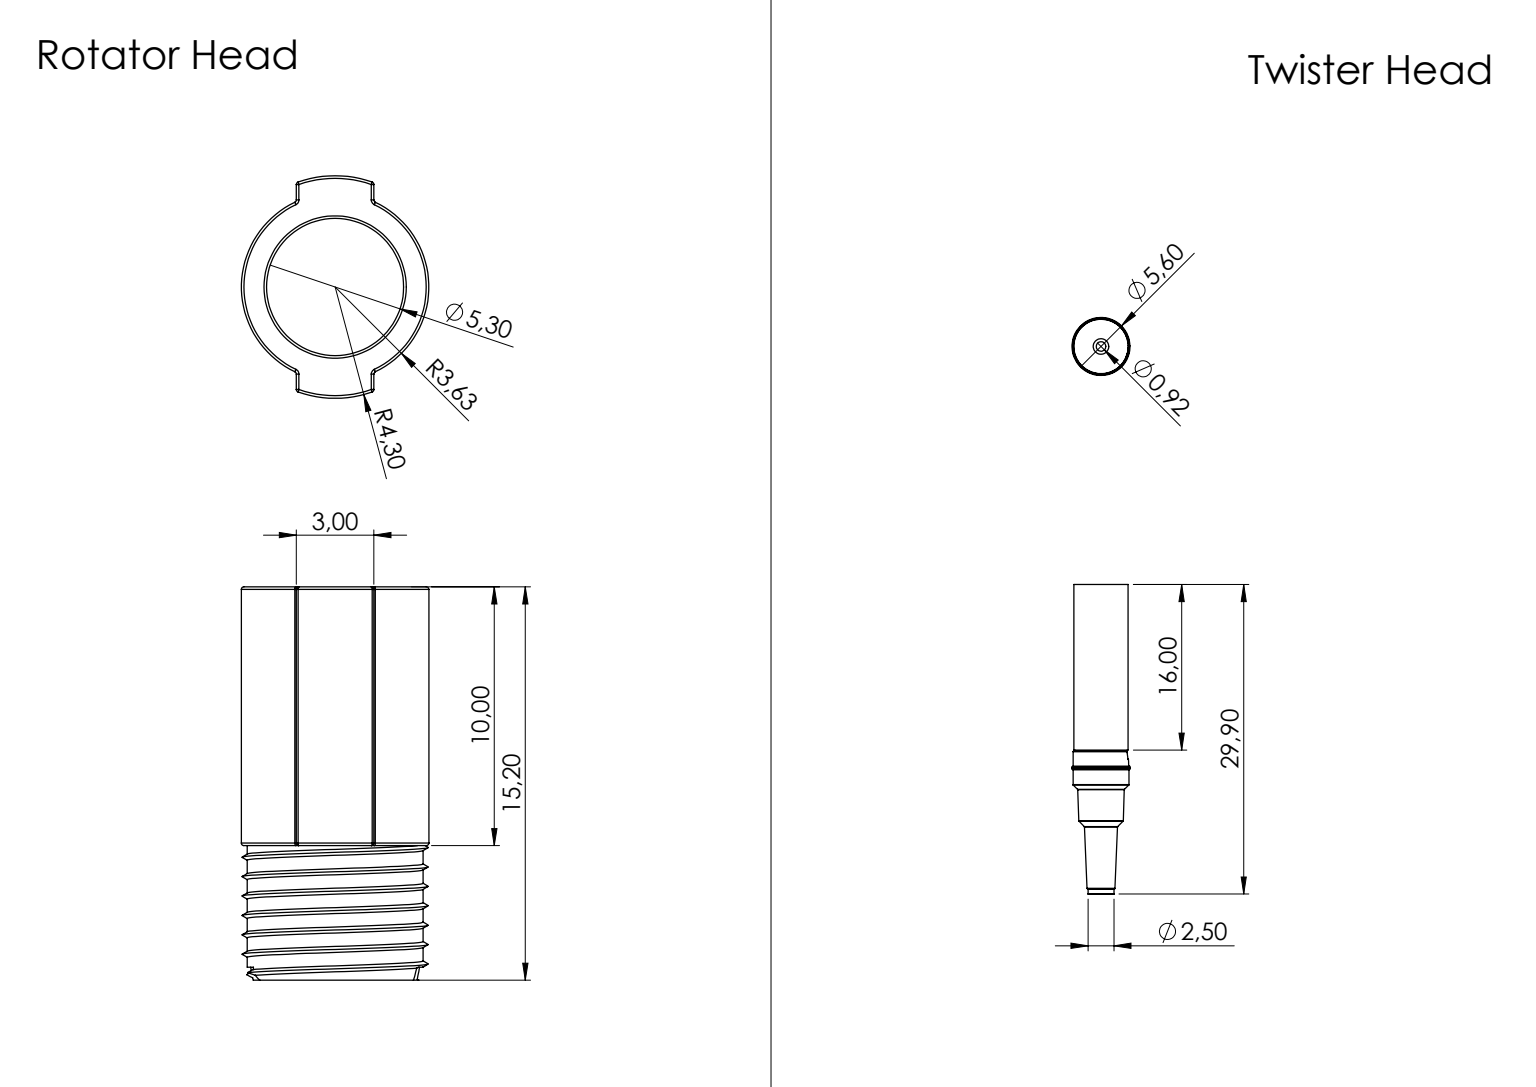
ISO-10303-21;
HEADER;
FILE_DESCRIPTION (('STEP AP214'),
    '1' );
FILE_NAME ('Twister Head.step',
    '2026-10-06T14:00:01',
    ( '' ),
    ( '' ),
    'SwSTEP 2.0',
    'SolidWorks 2020',
    '' );
FILE_SCHEMA (( 'AUTOMOTIVE_DESIGN' ));
ENDSEC;

DATA;
#8=CARTESIAN_POINT ( 'NONE',  ( -62.06147329307218286, -2.678446930503585843, 0.2197408810668839418 ) ) ;
#55=AXIS2_PLACEMENT_3D ( 'NONE', #1109, #22822, #12810 ) ;
#66=VERTEX_POINT ( 'NONE', #447 ) ;
#74=DIRECTION ( 'NONE',  ( -1.000000000000000000, -3.053848253006669023E-16, 2.042510438544995415E-16 ) ) ;
#122=DIRECTION ( 'NONE',  ( 3.002035892788117459E-16, -0.9996898646859343485, -0.02490330187381124480 ) ) ;
#150=CARTESIAN_POINT ( 'NONE',  ( -61.38060080783325390, -2.623833477274086334, -0.6199702340732970995 ) ) ;
#158=DIRECTION ( 'NONE',  ( -1.000000000000000000, -3.053848253006669023E-16, 2.042510438544995415E-16 ) ) ;
#169=DIRECTION ( 'NONE',  ( 0.000000000000000000, -0.9996898646859343485, -0.02490330187381124133 ) ) ;
#190=CARTESIAN_POINT ( 'NONE',  ( -61.37597047653181903, -2.565398393854171122, -0.8228970461733545738 ) ) ;
#193=DIRECTION ( 'NONE',  ( 0.9994629430332292452, 0.03275911391080331414, 0.0008160631928537054542 ) ) ;
#221=ORIENTED_EDGE ( 'NONE', *, *, #12347, .T. ) ;
#253=ORIENTED_EDGE ( 'NONE', *, *, #12134, .F. ) ;
#254=CIRCLE ( 'NONE', #19476, 1.260000000000000231 ) ;
#306=DIRECTION ( 'NONE',  ( 1.000000000000000000, 3.053848253006669023E-16, -2.042510438544995415E-16 ) ) ;
#347=( GEOMETRIC_REPRESENTATION_CONTEXT ( 3 ) GLOBAL_UNCERTAINTY_ASSIGNED_CONTEXT ( ( #22477 ) ) GLOBAL_UNIT_ASSIGNED_CONTEXT ( ( #9070, #19057, #4625 ) ) REPRESENTATION_CONTEXT ( 'NONE', 'WORKASPACE' ) );
#395=EDGE_CURVE ( 'NONE', #29448, #3131, #5108, .T. ) ;
#418=CARTESIAN_POINT ( 'NONE',  ( -73.89999999999997726, 0.4598573377555273400, 0.01145551886195788835 ) ) ;
#427=EDGE_CURVE ( 'NONE', #3316, #29448, #13185, .T. ) ;
#434=ORIENTED_EDGE ( 'NONE', *, *, #19502, .F. ) ;
#447=CARTESIAN_POINT ( 'NONE',  ( -74.39999999999997726, -0.4598573377555325026, -0.01145551886194846360 ) ) ;
#449=FACE_OUTER_BOUND ( 'NONE', #30131, .T. ) ;
#500=CARTESIAN_POINT ( 'NONE',  ( -61.38648119981476015, -2.567347173575106556, -0.8311979704516511136 ) ) ;
#503=CARTESIAN_POINT ( 'NONE',  ( -62.09267578295094125, -2.518691627519130449, 0.1783745650731504706 ) ) ;
#514=CARTESIAN_POINT ( 'NONE',  ( -61.35318038805866081, -2.627373316876406850, 0.4646149771581839505 ) ) ;
#517=CARTESIAN_POINT ( 'NONE',  ( -67.32861504302871936, -2.100022785575387463, -0.05231372570481371970 ) ) ;
#580=CARTESIAN_POINT ( 'NONE',  ( -61.34999999999997300, -2.577403337407089712, -0.5873456857003641618 ) ) ;
#604=LINE ( 'NONE', #19783, #5091 ) ;
#626=CARTESIAN_POINT ( 'NONE',  ( -73.89999999999997726, 0.03361945752964275169, -1.349581317326006946 ) ) ;
#636=CARTESIAN_POINT ( 'NONE',  ( -61.34999999999997300, -2.603451079269508917, 0.4582852780074869736 ) ) ;
#648=CARTESIAN_POINT ( 'NONE',  ( -61.34999999999997300, -2.533482711517546893, -0.7936709607354018869 ) ) ;
#661=CARTESIAN_POINT ( 'NONE',  ( -61.39708522154533199, -2.653109165506343903, 0.5005920380465845865 ) ) ;
#668=ORIENTED_EDGE ( 'NONE', *, *, #22922, .F. ) ;
#680=ORIENTED_EDGE ( 'NONE', *, *, #27825, .F. ) ;
#685=CARTESIAN_POINT ( 'NONE',  ( -67.32861504302871936, -4.287230892216076523E-16, 3.265676834553754426E-15 ) ) ;
#702=CARTESIAN_POINT ( 'NONE',  ( -61.38483210406819524, -2.605333280927485173, 0.7010916910920483858 ) ) ;
#707=DIRECTION ( 'NONE',  ( 3.002035892788117952E-16, -0.9996898646859344595, -0.02490330187381124133 ) ) ;
#761=ORIENTED_EDGE ( 'NONE', *, *, #2889, .F. ) ;
#762=CARTESIAN_POINT ( 'NONE',  ( -61.34999999999997300, -2.456456838093036055, -0.5843327841101846332 ) ) ;
#766=DIRECTION ( 'NONE',  ( 0.7071067811865440200, -0.7068874824028898995, -0.01760929362890773994 ) ) ;
#775=EDGE_CURVE ( 'NONE', #13383, #3831, #22467, .T. ) ;
#782=FACE_OUTER_BOUND ( 'NONE', #5822, .T. ) ;
#784=CARTESIAN_POINT ( 'NONE',  ( -61.39999999999998437, 1.381785979968628826E-15, 2.054751023403646402E-15 ) ) ;
#790=DIRECTION ( 'NONE',  ( 1.000000000000000000, 3.053848253006669023E-16, -2.042510438544995415E-16 ) ) ;
#804=CARTESIAN_POINT ( 'NONE',  ( -67.32861504302871936, 2.100022785575386575, 0.05231372570482049900 ) ) ;
#814=ORIENTED_EDGE ( 'NONE', *, *, #5611, .F. ) ;
#851=EDGE_CURVE ( 'NONE', #22580, #19955, #11332, .T. ) ;
#866=ADVANCED_FACE ( 'NONE', ( #1077 ), #1719, .T. ) ;
#884=ORIENTED_EDGE ( 'NONE', *, *, #22321, .T. ) ;
#886=AXIS2_PLACEMENT_3D ( 'NONE', #30658, #14191, #19131 ) ;
#940=CARTESIAN_POINT ( 'NONE',  ( -62.06710100716626499, -2.504070139480777613, -0.3244344873171103316 ) ) ;
#942=FACE_OUTER_BOUND ( 'NONE', #27423, .T. ) ;
#966=CARTESIAN_POINT ( 'NONE',  ( -61.34999999999997300, -2.606726380931868370, 0.4585432435923214589 ) ) ;
#1017=DIRECTION ( 'NONE',  ( 0.000000000000000000, -0.9996898646859344595, -0.02490330187381124133 ) ) ;
#1069=CARTESIAN_POINT ( 'NONE',  ( -64.28602961791190751, 5.004363292900432036E-16, 2.644225585457161048E-15 ) ) ;
#1077=FACE_OUTER_BOUND ( 'NONE', #10203, .T. ) ;
#1088=CYLINDRICAL_SURFACE ( 'NONE', #11933, 0.7500000000000002220 ) ;
#1104=CYLINDRICAL_SURFACE ( 'NONE', #22252, 2.700000000000000178 ) ;
#1109=CARTESIAN_POINT ( 'NONE',  ( -73.90999999999998238, 1.259609229504275341, 0.03137816036100692790 ) ) ;
#1150=EDGE_CURVE ( 'NONE', #24563, #7611, #31047, .T. ) ;
#1172=CIRCLE ( 'NONE', #8246, 2.700000000000000178 ) ;
#1175=CARTESIAN_POINT ( 'NONE',  ( -61.39062294604998016, -2.605675279217121165, 0.7053491114958538866 ) ) ;
#1179=ORIENTED_EDGE ( 'NONE', *, *, #26385, .F. ) ;
#1180=FACE_OUTER_BOUND ( 'NONE', #3898, .T. ) ;
#1194=AXIS2_PLACEMENT_3D ( 'NONE', #4886, #26749, #24363 ) ;
#1217=ADVANCED_FACE ( 'NONE', ( #3874 ), #26027, .F. ) ;
#1234=ADVANCED_FACE ( 'NONE', ( #1498, #8931 ), #11007, .F. ) ;
#1253=EDGE_CURVE ( 'NONE', #13929, #13516, #22274, .T. ) ;
#1262=DIRECTION ( 'NONE',  ( 0.000000000000000000, 0.9996898646859343485, 0.02490330187381130031 ) ) ;
#1271=CARTESIAN_POINT ( 'NONE',  ( -62.06272861537543406, -2.661683864372939468, -0.3480657431877479668 ) ) ;
#1280=CARTESIAN_POINT ( 'NONE',  ( -60.64999999999998437, -2.458515422985869670, -1.116110171506649040 ) ) ;
#1290=PRESENTATION_STYLE_ASSIGNMENT (( #20643 ) ) ;
#1307=CARTESIAN_POINT ( 'NONE',  ( -64.31974649313019654, 2.248654970328750835, 0.05601630617085266717 ) ) ;
#1309=DIRECTION ( 'NONE',  ( 0.000000000000000000, 0.9996898646859344595, 0.02490330187381124133 ) ) ;
#1310=FACE_OUTER_BOUND ( 'NONE', #11555, .T. ) ;
#1315=DIRECTION ( 'NONE',  ( 1.000000000000000000, 3.053848253006669023E-16, -2.042510438544995415E-16 ) ) ;
#1321=B_SPLINE_CURVE_WITH_KNOTS ( 'NONE', 3,
 ( #22697, #3197, #20473, #20634, #27889, #13161, #20322, #22847, #29952, #13300, #30264, #17780, #15236, #22372, #3664, #6059, #15711, #30094, #1280 ),
 .UNSPECIFIED., .F., .F.,
 ( 4, 3, 3, 3, 3, 3, 4 ),
 ( 0.000000000000000000, 1.471960608404959728E-05, 2.936908138775533325E-05, 4.497395798386097826E-05, 6.315917083330272743E-05, 8.519491945895639831E-05, 8.667572485204743640E-05 ),
 .UNSPECIFIED. ) ;
#1325=CARTESIAN_POINT ( 'NONE',  ( -67.92156587216960872, -6.098012745906804249E-16, 3.386787660360170602E-15 ) ) ;
#1373=ORIENTED_EDGE ( 'NONE', *, *, #24338, .T. ) ;
#1402=EDGE_CURVE ( 'NONE', #22270, #22436, #30762, .T. ) ;
#1404=ORIENTED_EDGE ( 'NONE', *, *, #14756, .T. ) ;
#1432=CARTESIAN_POINT ( 'NONE',  ( -62.09999999999997300, -2.719773892260283876, -0.3638560033992588316 ) ) ;
#1473=ADVANCED_FACE ( 'NONE', ( #23597 ), #7274, .F. ) ;
#1481=MECHANICAL_DESIGN_GEOMETRIC_PRESENTATION_REPRESENTATION('',(#27754),#17683);
#1492=CIRCLE ( 'NONE', #26293, 2.685355339059328106 ) ;
#1498=FACE_OUTER_BOUND ( 'NONE', #11151, .T. ) ;
#1500=DIRECTION ( 'NONE',  ( -1.000000000000000000, -3.053848253006669023E-16, 2.042510438544995415E-16 ) ) ;
#1504=CARTESIAN_POINT ( 'NONE',  ( -61.34999999999997300, -2.482504579955461477, 0.4612981795977083577 ) ) ;
#1515=ORIENTED_EDGE ( 'NONE', *, *, #1253, .F. ) ;
#1527=DIRECTION ( 'NONE',  ( 0.000000000000000000, -0.9996898646859343485, -0.02490330187381124133 ) ) ;
#1529=CARTESIAN_POINT ( 'NONE',  ( -62.39999999999998437, 1.076401154667962023E-15, 2.259002067258145746E-15 ) ) ;
#1570=CARTESIAN_POINT ( 'NONE',  ( -62.09999999999998010, -2.737158043526072504, 0.2654540351181892688 ) ) ;
#1610=CARTESIAN_POINT ( 'NONE',  ( -60.49999999999997868, 2.624185894800580066, 0.06537116741875639847 ) ) ;
#1618=PLANE ( 'NONE',  #2300 ) ;
#1635=VERTEX_POINT ( 'NONE', #12633 ) ;
#1638=DIRECTION ( 'NONE',  ( 2.117927888850091331E-16, -0.02490330187381135929, 0.9996898646859343485 ) ) ;
#1641=VERTEX_POINT ( 'NONE', #10117 ) ;
#1659=ORIENTED_EDGE ( 'NONE', *, *, #1892, .T. ) ;
#1675=ORIENTED_EDGE ( 'NONE', *, *, #851, .F. ) ;
#1676=CARTESIAN_POINT ( 'NONE',  ( -73.89999999999997726, -0.7497673985144535092, -0.01867747640535382878 ) ) ;
#1677=FACE_OUTER_BOUND ( 'NONE', #21892, .T. ) ;
#1699=TOROIDAL_SURFACE ( 'NONE', #19434, 2.649999999999999911, 0.05000000000000000278 ) ;
#1702=ADVANCED_FACE ( 'NONE', ( #23094 ), #18343, .F. ) ;
#1704=ORIENTED_EDGE ( 'NONE', *, *, #29407, .F. ) ;
#1714=CARTESIAN_POINT ( 'NONE',  ( -61.39919398045554999, -2.624618644152858948, -0.6335224862127015744 ) ) ;
#1719=TOROIDAL_SURFACE ( 'NONE', #5786, 2.750000000000000000, 0.05000000000000000278 ) ;
#1732=DIRECTION ( 'NONE',  ( 0.000000000000000000, 0.9996898646859344595, 0.02490330187381105745 ) ) ;
#1734=VERTEX_POINT ( 'NONE', #3753 ) ;
#1735=CARTESIAN_POINT ( 'NONE',  ( -74.39999999999997726, 1.239615432210556367, 0.03088009432353080660 ) ) ;
#1760=EDGE_LOOP ( 'NONE', ( #12970, #14626, #2969, #14426 ) ) ;
#1799=DIRECTION ( 'NONE',  ( -1.000000000000000000, -3.053848253006669023E-16, 2.042510438544995169E-16 ) ) ;
#1803=CYLINDRICAL_SURFACE ( 'NONE', #15773, 2.625000000000000444 ) ;
#1808=VERTEX_POINT ( 'NONE', #13682 ) ;
#1827=VERTEX_POINT ( 'NONE', #6575 ) ;
#1831=VERTEX_POINT ( 'NONE', #1504 ) ;
#1843=FACE_BOUND ( 'NONE', #20133, .T. ) ;
#1845=ORIENTED_EDGE ( 'NONE', *, *, #7926, .T. ) ;
#1885=AXIS2_PLACEMENT_3D ( 'NONE', #11670, #28126, #16410 ) ;
#1892=EDGE_CURVE ( 'NONE', #3863, #2409, #3845, .T. ) ;
#1898=CARTESIAN_POINT ( 'NONE',  ( -62.09999999999998721, -2.677618807081935781, 0.1824170939552585136 ) ) ;
#1899=AXIS2_PLACEMENT_3D ( 'NONE', #11192, #13560, #3744 ) ;
#1903=CIRCLE ( 'NONE', #21669, 2.150647426004269835 ) ;
#1959=ORIENTED_EDGE ( 'NONE', *, *, #24978, .F. ) ;
#1979=DIRECTION ( 'NONE',  ( 1.000000000000000000, 3.053848253006669023E-16, -2.042510438544995415E-16 ) ) ;
#1982=AXIS2_PLACEMENT_3D ( 'NONE', #17687, #3261, #22592 ) ;
#2005=CIRCLE ( 'NONE', #18203, 2.700000000000000178 ) ;
#2027=CARTESIAN_POINT ( 'NONE',  ( -67.91948434493399134, -1.598692187574555446, -0.03982506530960670810 ) ) ;
#2030=ORIENTED_EDGE ( 'NONE', *, *, #6783, .F. ) ;
#2037=AXIS2_PLACEMENT_3D ( 'NONE', #3711, #15896, #25554 ) ;
#2039=DIRECTION ( 'NONE',  ( 1.000000000000000000, 3.053848253006669023E-16, -2.042510438544995415E-16 ) ) ;
#2073=ORIENTED_EDGE ( 'NONE', *, *, #11797, .T. ) ;
#2074=EDGE_CURVE ( 'NONE', #19955, #5910, #15898, .T. ) ;
#2079=ORIENTED_EDGE ( 'NONE', *, *, #30465, .T. ) ;
#2097=CARTESIAN_POINT ( 'NONE',  ( -60.84461143194913291, -2.333522038737472215, -0.9693817630866828905 ) ) ;
#2099=ORIENTED_EDGE ( 'NONE', *, *, #13067, .F. ) ;
#2101=EDGE_CURVE ( 'NONE', #21049, #9458, #14244, .T. ) ;
#2110=DIRECTION ( 'NONE',  ( 0.000000000000000000, -0.9996898646859344595, -0.02490330187381124133 ) ) ;
#2129=CARTESIAN_POINT ( 'NONE',  ( -62.09999999999997300, -2.678008572308610002, 0.1572561257273979995 ) ) ;
#2179=EDGE_LOOP ( 'NONE', ( #21179, #29517, #30612, #21844 ) ) ;
#2187=DIRECTION ( 'NONE',  ( -1.000000000000000000, -3.053848253006669023E-16, 2.042510438544995415E-16 ) ) ;
#2192=CIRCLE ( 'NONE', #25448, 2.525000000000001243 ) ;
#2197=CARTESIAN_POINT ( 'NONE',  ( -61.36380732660158799, -2.615533412885217679, -0.6059315537932544737 ) ) ;
#2206=B_SPLINE_CURVE_WITH_KNOTS ( 'NONE', 3,
 ( #22940, #20578, #10593, #22468, #24832, #19939, #8061, #7891, #27687, #29573, #3471, #3148, #13109, #12788, #8210, #13398, #6006, #17727, #20419 ),
 .UNSPECIFIED., .F., .F.,
 ( 4, 3, 3, 3, 3, 3, 4 ),
 ( 0.000000000000000000, 1.471960608404945498E-05, 2.936908138775499782E-05, 4.497395798386056491E-05, 6.315917083330130442E-05, 8.519491945895780777E-05, 8.667572485204612181E-05 ),
 .UNSPECIFIED. ) ;
#2208=EDGE_CURVE ( 'NONE', #4977, #1831, #29745, .T. ) ;
#2209=CARTESIAN_POINT ( 'NONE',  ( -61.58550117504142918, -2.616993147716194290, 0.3722059216910014179 ) ) ;
#2213=CARTESIAN_POINT ( 'NONE',  ( -62.06826892193116407, -2.655650422564618474, -0.3277852898564783124 ) ) ;
#2240=CARTESIAN_POINT ( 'NONE',  ( -60.59999999999997300, -2.458552378503722657, 0.9390651652154902163 ) ) ;
#2243=CARTESIAN_POINT ( 'NONE',  ( -60.59540624230464090, -2.407984592044280614, -1.061968112081668192 ) ) ;
#2250=DIRECTION ( 'NONE',  ( 0.000000000000000000, -0.9996898646859343485, -0.02490330187381143562 ) ) ;
#2271=ORIENTED_EDGE ( 'NONE', *, *, #7399, .F. ) ;
#2286=CARTESIAN_POINT ( 'NONE',  ( -60.59999999999997300, -2.471065902200942688, 0.9400020572919363104 ) ) ;
#2300=AXIS2_PLACEMENT_3D ( 'NONE', #28066, #25857, #6384 ) ;
#2378=CARTESIAN_POINT ( 'NONE',  ( -62.06395008846758543, -2.671759355462868246, 0.2104784954680237186 ) ) ;
#2409=VERTEX_POINT ( 'NONE', #2240 ) ;
#2421=AXIS2_PLACEMENT_3D ( 'NONE', #17430, #7625, #12521 ) ;
#2441=ORIENTED_EDGE ( 'NONE', *, *, #29407, .T. ) ;
#2443=EDGE_LOOP ( 'NONE', ( #12858, #26263, #19765, #17088 ) ) ;
#2459=DIRECTION ( 'NONE',  ( 0.000000000000000000, 0.02490330187380867394, -0.9996898646859344595 ) ) ;
#2467=VERTEX_POINT ( 'NONE', #10624 ) ;
#2484=FACE_OUTER_BOUND ( 'NONE', #7910, .T. ) ;
#2488=VERTEX_POINT ( 'NONE', #3026 ) ;
#2490=EDGE_CURVE ( 'NONE', #9458, #22270, #17710, .T. ) ;
#2506=CARTESIAN_POINT ( 'NONE',  ( -63.84999999999997300, 2.699162634652023662, 0.06723891505929292800 ) ) ;
#2509=ORIENTED_EDGE ( 'NONE', *, *, #23253, .T. ) ;
#2510=DIRECTION ( 'NONE',  ( 0.000000000000000000, 0.9996898646859347926, 0.02490330187379526453 ) ) ;
#2540=CARTESIAN_POINT ( 'NONE',  ( -62.05037051514401014, -2.687515796301105819, 0.2593462970732348660 ) ) ;
#2564=ORIENTED_EDGE ( 'NONE', *, *, #10095, .F. ) ;
#2594=VERTEX_POINT ( 'NONE', #8849 ) ;
#2600=DIRECTION ( 'NONE',  ( 1.000000000000000000, 3.053848253006669023E-16, -2.042510438544995415E-16 ) ) ;
#2611=CARTESIAN_POINT ( 'NONE',  ( -60.59999999999997300, -2.476825173781434852, 0.9422510591782664591 ) ) ;
#2612=FACE_OUTER_BOUND ( 'NONE', #1760, .T. ) ;
#2635=ORIENTED_EDGE ( 'NONE', *, *, #15008, .F. ) ;
#2647=ORIENTED_EDGE ( 'NONE', *, *, #775, .T. ) ;
#2670=FACE_OUTER_BOUND ( 'NONE', #24696, .T. ) ;
#2672=ORIENTED_EDGE ( 'NONE', *, *, #29379, .F. ) ;
#2700=ORIENTED_EDGE ( 'NONE', *, *, #3749, .F. ) ;
#2721=CARTESIAN_POINT ( 'NONE',  ( -61.39878663427906247, -2.566070302374152678, -0.8397640680202698160 ) ) ;
#2735=CARTESIAN_POINT ( 'NONE',  ( -61.37024607392400810, -2.647295961725869784, 0.4804220770584431977 ) ) ;
#2737=CIRCLE ( 'NONE', #25485, 2.150647426004269835 ) ;
#2834=CARTESIAN_POINT ( 'NONE',  ( -73.85208152723558328, -2.420890761855879333E-15, 4.598101673502850081E-15 ) ) ;
#2866=ORIENTED_EDGE ( 'NONE', *, *, #3749, .T. ) ;
#2876=MECHANICAL_DESIGN_GEOMETRIC_PRESENTATION_REPRESENTATION('',(#17530),#347);
#2878=CARTESIAN_POINT ( 'NONE',  ( -61.35350676116485857, -2.546188506968221521, -0.8003206670636398012 ) ) ;
#2889=EDGE_CURVE ( 'NONE', #3831, #19690, #27262, .T. ) ;
#2891=CARTESIAN_POINT ( 'NONE',  ( -61.36631426390781030, -2.644259247411960168, 0.4770650455704195658 ) ) ;
#2898=ORIENTED_EDGE ( 'NONE', *, *, #6137, .T. ) ;
#2901=VERTEX_POINT ( 'NONE', #27328 ) ;
#2905=EDGE_LOOP ( 'NONE', ( #26280, #1404, #23342, #680 ) ) ;
#2906=CARTESIAN_POINT ( 'NONE',  ( -44.49999999999997868, 6.542789527549899840E-15, -1.397091617737396343E-15 ) ) ;
#2907=CIRCLE ( 'NONE', #28164, 2.800000000000000266 ) ;
#2916=DIRECTION ( 'NONE',  ( 0.000000000000000000, -0.9996898646859344595, -0.02490330187381124133 ) ) ;
#2968=CARTESIAN_POINT ( 'NONE',  ( -60.59999999999997300, 2.524216908331986975, 0.06288083723137545544 ) ) ;
#2969=ORIENTED_EDGE ( 'NONE', *, *, #27825, .T. ) ;
#2980=ORIENTED_EDGE ( 'NONE', *, *, #7161, .T. ) ;
#2993=ORIENTED_EDGE ( 'NONE', *, *, #13490, .T. ) ;
#3012=PLANE ( 'NONE',  #15879 ) ;
#3014=VERTEX_POINT ( 'NONE', #23217 ) ;
#3026=CARTESIAN_POINT ( 'NONE',  ( -63.82928932188132620, 2.699162634652023662, 0.06723891505929291412 ) ) ;
#3032=CARTESIAN_POINT ( 'NONE',  ( -62.09999999999997300, -0.005353951483533918657, 0.2149229472152393294 ) ) ;
#3033=CARTESIAN_POINT ( 'NONE',  ( -61.35554497119343864, -2.549885958390812668, -0.8029968850693790516 ) ) ;
#3041=DIRECTION ( 'NONE',  ( 1.000000000000000000, 3.053848253006669023E-16, -2.042510438544995415E-16 ) ) ;
#3054=ORIENTED_EDGE ( 'NONE', *, *, #28349, .T. ) ;
#3074=TOROIDAL_SURFACE ( 'NONE', #21799, 2.299325721147392088, 0.05000000000000000278 ) ;
#3083=CARTESIAN_POINT ( 'NONE',  ( -62.08544523815352534, -2.505505003946113973, -0.3131916526553849556 ) ) ;
#3086=CARTESIAN_POINT ( 'NONE',  ( -60.84484350713346146, -2.494647975071613732, 0.8490225916460741873 ) ) ;
#3109=AXIS2_PLACEMENT_3D ( 'NONE', #8983, #13862, #18657 ) ;
#3131=VERTEX_POINT ( 'NONE', #3984 ) ;
#3137=DIRECTION ( 'NONE',  ( 3.002035892788117459E-16, -0.9996898646859343485, -0.02490330187381124480 ) ) ;
#3142=DIRECTION ( 'NONE',  ( 0.000000000000000000, 0.02490330187380866006, -0.9996898646859344595 ) ) ;
#3146=( BOUNDED_CURVE ( )  B_SPLINE_CURVE ( 3, ( #15173, #10115, #24825, #12941 ),
 .UNSPECIFIED., .F., .T. ) 
 B_SPLINE_CURVE_WITH_KNOTS ( ( 4, 4 ),
 ( 1.358646995387534862, 1.449211172151202653 ),
 .UNSPECIFIED. ) 
 CURVE ( )  GEOMETRIC_REPRESENTATION_ITEM ( )  RATIONAL_B_SPLINE_CURVE ( ( 1.000000000000000000, 0.9993166276053078168, 0.9993166276053078168, 1.000000000000000000 ) ) 
 REPRESENTATION_ITEM ( '' )  );
#3148=CARTESIAN_POINT ( 'NONE',  ( -60.62613029541262222, -2.511626612308461404, 0.9750051806848812896 ) ) ;
#3171=CARTESIAN_POINT ( 'NONE',  ( -61.34999999999997300, -2.600201727571727517, 0.4583662226975599441 ) ) ;
#3182=CARTESIAN_POINT ( 'NONE',  ( -63.82928932188132620, 6.399178848011186396E-16, 2.550935903222500290E-15 ) ) ;
#3196=CARTESIAN_POINT ( 'NONE',  ( -61.39623369212913673, -2.653156182710691535, 0.4999952066012984808 ) ) ;
#3197=CARTESIAN_POINT ( 'NONE',  ( -60.59999999999997300, -2.431313162469589173, -1.066416437073405499 ) ) ;
#3237=CARTESIAN_POINT ( 'NONE',  ( -62.09716160983483491, -2.507809103222365721, -0.2941402757104731314 ) ) ;
#3240=CARTESIAN_POINT ( 'NONE',  ( -61.39878663427906957, -2.604700304447900017, 0.7109548583936591282 ) ) ;
#3244=AXIS2_PLACEMENT_3D ( 'NONE', #7705, #29712, #19762 ) ;
#3261=DIRECTION ( 'NONE',  ( 1.000000000000000000, 3.053848253006669023E-16, -2.042510438544995415E-16 ) ) ;
#3266=CARTESIAN_POINT ( 'NONE',  ( -44.49999999999997868, -2.624185894800571628, -0.06537116741875388659 ) ) ;
#3288=FACE_OUTER_BOUND ( 'NONE', #18600, .T. ) ;
#3302=AXIS2_PLACEMENT_3D ( 'NONE', #5119, #10037, #14771 ) ;
#3311=EDGE_LOOP ( 'NONE', ( #22876, #22227, #28198, #5471, #29228, #20446, #8081, #17588 ) ) ;
#3316=VERTEX_POINT ( 'NONE', #26311 ) ;
#3330=AXIS2_PLACEMENT_3D ( 'NONE', #8769, #23215, #6259 ) ;
#3361=DIRECTION ( 'NONE',  ( -1.000000000000000000, -3.053848253006669023E-16, 2.042510438544995415E-16 ) ) ;
#3375=ORIENTED_EDGE ( 'NONE', *, *, #24341, .T. ) ;
#3388=DIRECTION ( 'NONE',  ( 1.000000000000000000, 3.053848253006669023E-16, -2.042510438544995415E-16 ) ) ;
#3440=AXIS2_PLACEMENT_3D ( 'NONE', #13751, #28344, #29282 ) ;
#3462=ORIENTED_EDGE ( 'NONE', *, *, #9789, .T. ) ;
#3465=CARTESIAN_POINT ( 'NONE',  ( -61.58692253671846828, -2.595286993531995545, -0.5015316826422865359 ) ) ;
#3471=CARTESIAN_POINT ( 'NONE',  ( -60.62155403265821718, -2.510184553012070552, 0.9710796741145765187 ) ) ;
#3478=DIRECTION ( 'NONE',  ( -1.000000000000000000, -3.053848253006669023E-16, 2.042510438544995415E-16 ) ) ;
#3504=PRODUCT_DEFINITION_FORMATION_WITH_SPECIFIED_SOURCE ( 'ANY', '', #16726, .NOT_KNOWN. ) ;
#3511=CARTESIAN_POINT ( 'NONE',  ( -60.59999999999998010, -2.408745774756101188, -1.060314564156378037 ) ) ;
#3542=CARTESIAN_POINT ( 'NONE',  ( -62.09999999999997300, 1.168016602258162478E-15, 2.197726754101795588E-15 ) ) ;
#3549=CARTESIAN_POINT ( 'NONE',  ( -73.89999999999997726, -2.435524336289708093E-15, 4.607889071584891164E-15 ) ) ;
#3574=CARTESIAN_POINT ( 'NONE',  ( -61.82615520548803545, -2.629528139897267192, 0.2842755848553404352 ) ) ;
#3582=CARTESIAN_POINT ( 'NONE',  ( -44.49999999999997868, 0.7497673985144576170, 0.01867747640535713169 ) ) ;
#3599=CARTESIAN_POINT ( 'NONE',  ( -61.39999999999998437, -2.565822298769830478, -0.8405688140393350327 ) ) ;
#3606=DIRECTION ( 'NONE',  ( 1.000000000000000000, 3.053848253006669023E-16, -2.042510438544995415E-16 ) ) ;
#3613=AXIS2_PLACEMENT_3D ( 'NONE', #12614, #27820, #22444 ) ;
#3646=DIRECTION ( 'NONE',  ( 0.000000000000000000, 0.9996898646859344595, 0.02490330187381124480 ) ) ;
#3664=CARTESIAN_POINT ( 'NONE',  ( -60.64271989919366490, -2.460423958995413773, -1.111508252306596001 ) ) ;
#3666=CARTESIAN_POINT ( 'NONE',  ( -61.39999999999998437, -2.624491116890564690, -0.6340712715164679159 ) ) ;
#3680=CARTESIAN_POINT ( 'NONE',  ( -61.58695197172909275, -2.498609834268938901, 0.3746267610600896858 ) ) ;
#3683=CARTESIAN_POINT ( 'NONE',  ( -73.89999999999997726, -2.435524336289708093E-15, 4.607889071584891164E-15 ) ) ;
#3711=CARTESIAN_POINT ( 'NONE',  ( -60.59999999999997300, 1.626093840209163176E-15, 1.891350188320046374E-15 ) ) ;
#3712=CARTESIAN_POINT ( 'NONE',  ( -62.09999999999997300, 1.168016602258162478E-15, 2.197726754101795588E-15 ) ) ;
#3725=DIRECTION ( 'NONE',  ( -1.000000000000000000, -3.053848253006669023E-16, 2.042510438544995415E-16 ) ) ;
#3744=DIRECTION ( 'NONE',  ( 0.000000000000000000, -0.9996898646859344595, -0.02490330187381133153 ) ) ;
#3749=EDGE_CURVE ( 'NONE', #28771, #23537, #16905, .T. ) ;
#3753=CARTESIAN_POINT ( 'NONE',  ( -67.88621053311027254, 1.613288973786557223, 0.04018868625473467210 ) ) ;
#3775=ADVANCED_FACE ( 'NONE', ( #12608 ), #29038, .T. ) ;
#3780=EDGE_CURVE ( 'NONE', #1641, #22580, #15100, .T. ) ;
#3783=ADVANCED_FACE ( 'NONE', ( #8603 ), #13837, .T. ) ;
#3803=CARTESIAN_POINT ( 'NONE',  ( -62.09999999999997300, -2.722123828016836722, -0.3761544999221376195 ) ) ;
#3812=AXIS2_PLACEMENT_3D ( 'NONE', #11235, #21247, #30544 ) ;
#3831=VERTEX_POINT ( 'NONE', #4160 ) ;
#3845=B_SPLINE_CURVE_WITH_KNOTS ( 'NONE', 3,
 ( #2611, #2286, #19563, #23986 ),
 .UNSPECIFIED., .F., .F.,
 ( 4, 4 ),
 ( 0.000000000000000000, 1.854844919671783956E-05 ),
 .UNSPECIFIED. ) ;
#3863=VERTEX_POINT ( 'NONE', #11921 ) ;
#3874=FACE_OUTER_BOUND ( 'NONE', #21190, .T. ) ;
#3879=AXIS2_PLACEMENT_3D ( 'NONE', #6964, #16449, #11703 ) ;
#3890=FACE_OUTER_BOUND ( 'NONE', #17344, .T. ) ;
#3898=EDGE_LOOP ( 'NONE', ( #13346, #29072, #6953, #9318 ) ) ;
#3924=AXIS2_PLACEMENT_3D ( 'NONE', #17146, #19518, #12672 ) ;
#3954=CARTESIAN_POINT ( 'NONE',  ( -60.64999999999998437, -2.458515422985869670, -1.116110171506649040 ) ) ;
#3967=DIRECTION ( 'NONE',  ( 1.000000000000000000, 3.053848253006669023E-16, -2.042510438544995415E-16 ) ) ;
#3971=CARTESIAN_POINT ( 'NONE',  ( -62.06697778907421537, -2.637963160708082899, -0.3297769518696585522 ) ) ;
#3976=ORIENTED_EDGE ( 'NONE', *, *, #6682, .T. ) ;
#3979=ADVANCED_FACE ( 'NONE', ( #5107 ), #19692, .T. ) ;
#3984=CARTESIAN_POINT ( 'NONE',  ( -73.89999999999997726, -1.259609229504280004, -0.03137816036099756040 ) ) ;
#4009=CARTESIAN_POINT ( 'NONE',  ( -73.84999999999996589, -2.420255095024673698E-15, 4.597676519392165349E-15 ) ) ;
#4010=CIRCLE ( 'NONE', #21746, 0.7500000000000002220 ) ;
#4071=DIRECTION ( 'NONE',  ( 0.000000000000000000, 0.9996898646859343485, 0.02490330187381123786 ) ) ;
#4102=ORIENTED_EDGE ( 'NONE', *, *, #19010, .F. ) ;
#4107=CARTESIAN_POINT ( 'NONE',  ( -61.39959699979583263, -2.624557268248721265, -0.6337974637291527991 ) ) ;
#4110=ORIENTED_EDGE ( 'NONE', *, *, #24246, .F. ) ;
#4120=CARTESIAN_POINT ( 'NONE',  ( -62.09999999999998010, -2.729213130609289717, -0.3426631772468137771 ) ) ;
#4132=ORIENTED_EDGE ( 'NONE', *, *, #25476, .F. ) ;
#4135=ORIENTED_EDGE ( 'NONE', *, *, #26385, .T. ) ;
#4140=SURFACE_STYLE_FILL_AREA ( #20938 ) ;
#4160=CARTESIAN_POINT ( 'NONE',  ( -62.09999999999997300, -2.737158043526071172, 0.2654540351181889912 ) ) ;
#4164=EDGE_CURVE ( 'NONE', #1808, #1734, #22433, .T. ) ;
#4170=ORIENTED_EDGE ( 'NONE', *, *, #6103, .F. ) ;
#4178=LINE ( 'NONE', #13816, #20768 ) ;
#4183=DIRECTION ( 'NONE',  ( 3.002035892788117459E-16, -0.9996898646859343485, -0.02490330187381124133 ) ) ;
#4184=CARTESIAN_POINT ( 'NONE',  ( -67.91948434493399134, -6.091656077594763675E-16, 3.386362506249485869E-15 ) ) ;
#4202=ORIENTED_EDGE ( 'NONE', *, *, #18602, .F. ) ;
#4215=DIRECTION ( 'NONE',  ( 0.000000000000000000, 0.9996898646859344595, 0.02490330187381124480 ) ) ;
#4216=CARTESIAN_POINT ( 'NONE',  ( -60.49999999999997868, 1.656632322739229403E-15, 1.870925083934595927E-15 ) ) ;
#4220=ADVANCED_FACE ( 'NONE', ( #13762 ), #4276, .T. ) ;
#4255=CARTESIAN_POINT ( 'NONE',  ( -61.34999999999997300, -2.583824419212624957, -0.5885162450438690129 ) ) ;
#4256=CARTESIAN_POINT ( 'NONE',  ( -62.34999999999997300, 2.749147127886321318, 0.06848408015298348972 ) ) ;
#4261=APPLICATION_CONTEXT ( 'automotive_design' ) ;
#4264=AXIS2_PLACEMENT_3D ( 'NONE', #13850, #30821, #1527 ) ;
#4270=CARTESIAN_POINT ( 'NONE',  ( -62.04999999999998295, -2.636465585633694264, 0.1493792525119592429 ) ) ;
#4274=CARTESIAN_POINT ( 'NONE',  ( -61.34999999999997300, -2.617575446388284099, 0.6620413751912884726 ) ) ;
#4276=CYLINDRICAL_SURFACE ( 'NONE', #29248, 2.525000000000001243 ) ;
#4282=AXIS2_PLACEMENT_3D ( 'NONE', #10523, #8596, #8444 ) ;
#4303=CARTESIAN_POINT ( 'NONE',  ( -60.85363833753338270, -2.450811742487699174, -0.9690170259278018117 ) ) ;
#4373=ORIENTED_EDGE ( 'NONE', *, *, #30925, .T. ) ;
#4379=AXIS2_PLACEMENT_3D ( 'NONE', #3542, #8130, #17802 ) ;
#4382=VECTOR ( 'NONE', #10935, 1000.000000000000000 ) ;
#4418=AXIS2_PLACEMENT_3D ( 'NONE', #3182, #27550, #13147 ) ;
#4431=VECTOR ( 'NONE', #6963, 1000.000000000000000 ) ;
#4432=DIRECTION ( 'NONE',  ( 1.000000000000000000, 3.053848253006669023E-16, -2.042510438544995415E-16 ) ) ;
#4446=CARTESIAN_POINT ( 'NONE',  ( -62.05783247874898478, -2.669955732903997792, -0.3664444735944112908 ) ) ;
#4504=( BOUNDED_SURFACE ( )  B_SPLINE_SURFACE ( 3, 2, ( 
 ( #16350, #19053, #4623 ),
 ( #26473, #30760, #11757 ),
 ( #7019, #14283, #4303 ),
 ( #28860, #4943, #2243 ) ),
 .UNSPECIFIED., .F., .F., .F. ) 
 B_SPLINE_SURFACE_WITH_KNOTS ( ( 4, 4 ),
 ( 3, 3 ),
 ( 5.003379805550770776, 5.119240129666620120 ),
 ( 0.000000000000000000, 1.000000000000000000 ),
 .UNSPECIFIED. ) 
 GEOMETRIC_REPRESENTATION_ITEM ( )  RATIONAL_B_SPLINE_SURFACE ( (
 ( 1.000000000000000000, 0.6043181045777066274, 1.000000000000000000),
 ( 1.000000000000000000, 0.5899361674293883695, 1.000000000000000000),
 ( 1.000000000000000000, 0.5752896509278045967, 1.000000000000000000),
 ( 1.000000000000000000, 0.5604218610591197303, 1.000000000000000000) ) ) 
 REPRESENTATION_ITEM ( '' )  SURFACE ( )  );
#4534=VERTEX_POINT ( 'NONE', #27225 ) ;
#4536=DIRECTION ( 'NONE',  ( 1.000000000000000000, 3.053848253006669023E-16, -2.042510438544995415E-16 ) ) ;
#4582=CARTESIAN_POINT ( 'NONE',  ( -61.35799158996540825, -2.608967300040148984, -0.6002010391711750659 ) ) ;
#4594=CARTESIAN_POINT ( 'NONE',  ( -62.09999999999998010, -2.625757682666624682, -0.2804666419185123383 ) ) ;
#4623=CARTESIAN_POINT ( 'NONE',  ( -61.38768957378469793, -2.520043259258192503, -0.7763025981709992251 ) ) ;
#4624=AXIS2_PLACEMENT_3D ( 'NONE', #14198, #4695, #26721 ) ;
#4625=( NAMED_UNIT ( * ) SI_UNIT ( $, .STERADIAN. ) SOLID_ANGLE_UNIT ( ) );
#4627=B_SPLINE_CURVE_WITH_KNOTS ( 'NONE', 3,
 ( #7882, #27211, #5522, #30317, #8625, #6886, #26032, #21321, #23838, #16385, #7055, #28264, #9595, #7204, #2129, #9269, #11791, #18932, #30623 ),
 .UNSPECIFIED., .F., .F.,
 ( 4, 3, 3, 3, 3, 3, 4 ),
 ( 0.000000000000000000, 6.909591911046148761E-06, 4.342671684267912936E-05, 7.786482953143393916E-05, 0.0001105775006590781824, 0.0001427429525918440115, 0.0001749426303720831523 ),
 .UNSPECIFIED. ) ;
#4628=DIRECTION ( 'NONE',  ( 2.117927888850091331E-16, -0.02490330187381135929, 0.9996898646859343485 ) ) ;
#4665=CARTESIAN_POINT ( 'NONE',  ( -61.39999999999998437, -2.604492677689918878, 0.7117709546332967596 ) ) ;
#4668=CARTESIAN_POINT ( 'NONE',  ( -60.49999999999997868, 1.656632322739229403E-15, 1.870925083934595927E-15 ) ) ;
#4669=CARTESIAN_POINT ( 'NONE',  ( -73.90999999999998238, -1.259609229504280004, -0.03137816036099756040 ) ) ;
#4670=B_SPLINE_CURVE_WITH_KNOTS ( 'NONE', 3,
 ( #25797, #4107, #1714, #13134, #20444, #23904, #150, #16635, #13900, #21540, #2197, #31016, #4582, #19174, #28338, #16785, #11860, #7267, #4255 ),
 .UNSPECIFIED., .F., .F.,
 ( 4, 3, 3, 3, 3, 3, 4 ),
 ( -1.475060283556113230E-06, 0.000000000000000000, 2.253555103675729373E-05, 4.073269212999672338E-05, 5.627305529011999768E-05, 7.083906737679824997E-05, 8.547717314343541571E-05 ),
 .UNSPECIFIED. ) ;
#4684=CARTESIAN_POINT ( 'NONE',  ( -67.89999999999997726, -6.032153844857049047E-16, 3.382382808457892732E-15 ) ) ;
#4685=ORIENTED_EDGE ( 'NONE', *, *, #25214, .F. ) ;
#4695=DIRECTION ( 'NONE',  ( 0.3420201433256656043, -0.02340144900402423012, 0.9394011889198369269 ) ) ;
#4710=VERTEX_POINT ( 'NONE', #8675 ) ;
#4723=DIRECTION ( 'NONE',  ( 0.000000000000000000, 0.9953301976458442946, -0.09652874004297590238 ) ) ;
#4733=CARTESIAN_POINT ( 'NONE',  ( -62.06576242361286688, -2.663271400516645127, 0.2033751180053996188 ) ) ;
#4737=FACE_OUTER_BOUND ( 'NONE', #30449, .T. ) ;
#4757=DIRECTION ( 'NONE',  ( -1.000000000000000000, -3.053848253006669023E-16, 2.042510438544995415E-16 ) ) ;
#4774=FACE_OUTER_BOUND ( 'NONE', #20120, .T. ) ;
#4783=ADVANCED_FACE ( 'NONE', ( #10569 ), #10713, .T. ) ;
#4848=CARTESIAN_POINT ( 'NONE',  ( -62.04999999999998295, 1.183285843523195887E-15, 2.187514201909070562E-15 ) ) ;
#4860=DIRECTION ( 'NONE',  ( -1.000000000000000000, -3.053848253006669023E-16, 2.042510438544995415E-16 ) ) ;
#4886=CARTESIAN_POINT ( 'NONE',  ( -63.82928932188132620, 6.399178848011186396E-16, 2.550935903222500290E-15 ) ) ;
#4901=CARTESIAN_POINT ( 'NONE',  ( -62.05303033788776190, -2.687940397879565513, 0.2501026294260040861 ) ) ;
#4903=CARTESIAN_POINT ( 'NONE',  ( -62.06974646775923787, -2.693531034594032203, 0.1939937330634021184 ) ) ;
#4907=CIRCLE ( 'NONE', #3812, 0.7500000000000002220 ) ;
#4935=AXIS2_PLACEMENT_3D ( 'NONE', #10870, #15473, #13382 ) ;
#4943=CARTESIAN_POINT ( 'NONE',  ( -60.58528264635176441, -2.480971988140598050, -1.067472133821737446 ) ) ;
#4977=VERTEX_POINT ( 'NONE', #24457 ) ;
#4990=FACE_OUTER_BOUND ( 'NONE', #23126, .T. ) ;
#5000=EDGE_LOOP ( 'NONE', ( #28846, #23493, #15348, #28122 ) ) ;
#5004=ORIENTED_EDGE ( 'NONE', *, *, #12849, .F. ) ;
#5021=DIRECTION ( 'NONE',  ( -1.000000000000000000, -3.053848253006669023E-16, 2.042510438544995415E-16 ) ) ;
#5024=ORIENTED_EDGE ( 'NONE', *, *, #24099, .T. ) ;
#5029=CARTESIAN_POINT ( 'NONE',  ( -61.39999999999998437, 1.381785979968628826E-15, 2.054751023403646402E-15 ) ) ;
#5035=FACE_OUTER_BOUND ( 'NONE', #12205, .T. ) ;
#5065=CARTESIAN_POINT ( 'NONE',  ( -67.36397038208805554, -2.135367159695522155, -0.05319419038625883972 ) ) ;
#5083=EDGE_CURVE ( 'NONE', #8829, #6950, #6154, .T. ) ;
#5085=VERTEX_POINT ( 'NONE', #22567 ) ;
#5091=VECTOR ( 'NONE', #20263, 1000.000000000000114 ) ;
#5101=DIRECTION ( 'NONE',  ( 0.000000000000000000, -0.9996898646859344595, -0.02490330187381124480 ) ) ;
#5104=DIRECTION ( 'NONE',  ( 0.9991330730923518866, 0.04161763361012259937, 0.001036738022138443578 ) ) ;
#5107=FACE_OUTER_BOUND ( 'NONE', #7591, .T. ) ;
#5108=CIRCLE ( 'NONE', #12186, 1.260000000000000231 ) ;
#5114=ADVANCED_FACE ( 'NONE', ( #8297 ), #30559, .T. ) ;
#5119=CARTESIAN_POINT ( 'NONE',  ( -67.92156587216960872, -1.648633347906702129, -0.04106915093617326262 ) ) ;
#5151=ADVANCED_FACE ( 'NONE', ( #13511 ), #24007, .T. ) ;
#5171=FACE_OUTER_BOUND ( 'NONE', #10876, .T. ) ;
#5195=DIRECTION ( 'NONE',  ( 0.7071067811865435759, 0.7068874824028903436, 0.01760929362890753525 ) ) ;
#5224=FACE_OUTER_BOUND ( 'NONE', #25462, .T. ) ;
#5265=ORIENTED_EDGE ( 'NONE', *, *, #5279, .F. ) ;
#5279=EDGE_CURVE ( 'NONE', #3014, #14583, #29798, .T. ) ;
#5282=AXIS2_PLACEMENT_3D ( 'NONE', #11513, #11330, #23388 ) ;
#5296=AXIS2_PLACEMENT_3D ( 'NONE', #7134, #158, #14713 ) ;
#5330=CARTESIAN_POINT ( 'NONE',  ( -61.34138888940498902, -2.634947490092511835, -0.5919143299442317652 ) ) ;
#5367=ORIENTED_EDGE ( 'NONE', *, *, #30465, .F. ) ;
#5369=AXIS2_PLACEMENT_3D ( 'NONE', #5614, #15263, #24910 ) ;
#5387=ADVANCED_FACE ( 'NONE', ( #27704, #27860 ), #13268, .F. ) ;
#5410=TOROIDAL_SURFACE ( 'NONE', #16548, 2.100674278852607824, 0.05000000000000000278 ) ;
#5414=CARTESIAN_POINT ( 'NONE',  ( -62.09999999999997300, -2.652521544886486726, -0.2850577375623332688 ) ) ;
#5418=AXIS2_PLACEMENT_3D ( 'NONE', #11222, #15681, #20896 ) ;
#5441=EDGE_CURVE ( 'NONE', #18442, #24092, #12117, .T. ) ;
#5454=ADVANCED_FACE ( 'NONE', ( #24994 ), #1104, .T. ) ;
#5466=CARTESIAN_POINT ( 'NONE',  ( -62.09902692368709154, -2.508428807930398019, -0.2888567384445905328 ) ) ;
#5470=ORIENTED_EDGE ( 'NONE', *, *, #10588, .F. ) ;
#5471=ORIENTED_EDGE ( 'NONE', *, *, #16202, .F. ) ;
#5498=ORIENTED_EDGE ( 'NONE', *, *, #13248, .F. ) ;
#5504=CARTESIAN_POINT ( 'NONE',  ( -61.82790928944205433, -2.612260643635529345, -0.4142152978364393445 ) ) ;
#5514=CARTESIAN_POINT ( 'NONE',  ( -62.14999999999998437, 1.152747360993128871E-15, 2.207939306294521009E-15 ) ) ;
#5522=CARTESIAN_POINT ( 'NONE',  ( -62.09999999999997300, -2.737532885411323669, 0.2608613065085638727 ) ) ;
#5527=DIRECTION ( 'NONE',  ( -1.000000000000000000, -3.053848253006669023E-16, 2.042510438544995415E-16 ) ) ;
#5530=EDGE_CURVE ( 'NONE', #7506, #28771, #6961, .T. ) ;
#5536=CARTESIAN_POINT ( 'NONE',  ( -73.89999999999997726, -2.435524336289708093E-15, 4.607889071584891164E-15 ) ) ;
#5569=LINE ( 'NONE', #3032, #30204 ) ;
#5571=EDGE_CURVE ( 'NONE', #30944, #13383, #2005, .T. ) ;
#5585=CARTESIAN_POINT ( 'NONE',  ( -61.39999999999998437, -2.652806974455509170, 0.5026083527760007996 ) ) ;
#5611=EDGE_CURVE ( 'NONE', #14068, #11253, #4010, .T. ) ;
#5614=CARTESIAN_POINT ( 'NONE',  ( -62.04999999999998295, 0.005353951483536231043, -0.2149229472152333897 ) ) ;
#5625=CARTESIAN_POINT ( 'NONE',  ( -61.35067641704169006, -2.574083687496825590, 0.6681602693401289539 ) ) ;
#5633=CARTESIAN_POINT ( 'NONE',  ( -62.06710100716626499, -2.504070139480777613, -0.3244344873171103316 ) ) ;
#5644=CARTESIAN_POINT ( 'NONE',  ( -61.82078168762245696, -2.687023538218675345, 0.2847997227030995560 ) ) ;
#5686=DIRECTION ( 'NONE',  ( -2.117927888850090838E-16, 0.02490330187381123786, -0.9996898646859343485 ) ) ;
#5696=DIRECTION ( 'NONE',  ( 0.000000000000000000, 0.9996898646859344595, 0.02490330187381124133 ) ) ;
#5754=DIRECTION ( 'NONE',  ( 3.002035892788117459E-16, -0.9996898646859344595, -0.02490330187381124133 ) ) ;
#5774=CARTESIAN_POINT ( 'NONE',  ( -61.39959552429773737, -2.604566667188200846, 0.7115002142985770162 ) ) ;
#5777=AXIS2_PLACEMENT_3D ( 'NONE', #26484, #31247, #11279 ) ;
#5786=AXIS2_PLACEMENT_3D ( 'NONE', #27835, #24824, #3137 ) ;
#5817=CARTESIAN_POINT ( 'NONE',  ( -62.09999999999997300, 2.749147127886321318, 0.06848408015298343421 ) ) ;
#5821=AXIS2_PLACEMENT_3D ( 'NONE', #517, #10173, #15084 ) ;
#5822=EDGE_LOOP ( 'NONE', ( #25678, #16377 ) ) ;
#5844=DIRECTION ( 'NONE',  ( 0.000000000000000000, -0.9996898646859343485, -0.02490330187381124133 ) ) ;
#5852=VERTEX_POINT ( 'NONE', #5817 ) ;
#5858=DIRECTION ( 'NONE',  ( -3.002035892788116966E-16, 0.9996898646859343485, 0.02490330187381123786 ) ) ;
#5863=AXIS2_PLACEMENT_3D ( 'NONE', #8279, #10806, #5754 ) ;
#5877=EDGE_CURVE ( 'NONE', #6272, #23465, #26694, .T. ) ;
#5878=CARTESIAN_POINT ( 'NONE',  ( -61.34999999999997300, -2.600201727571727517, 0.4583662226975599441 ) ) ;
#5882=DIRECTION ( 'NONE',  ( -3.002035892788117459E-16, 0.9996898646859344595, 0.02490330187381124133 ) ) ;
#5905=( LENGTH_UNIT ( ) NAMED_UNIT ( * ) SI_UNIT ( .MILLI., .METRE. ) );
#5910=VERTEX_POINT ( 'NONE', #20558 ) ;
#5915=AXIS2_PLACEMENT_3D ( 'NONE', #11872, #11571, #23767 ) ;
#5942=DIRECTION ( 'NONE',  ( 0.000000000000000000, 0.9996898646859343485, 0.02490330187381123786 ) ) ;
#5962=CARTESIAN_POINT ( 'NONE',  ( -74.39999999999997726, -2.588216748940040213E-15, 4.710014593512140639E-15 ) ) ;
#5969=CARTESIAN_POINT ( 'NONE',  ( -60.61250724947092294, -2.505441611314725314, 1.006360935396775069 ) ) ;
#6006=CARTESIAN_POINT ( 'NONE',  ( -60.64918514029854180, -2.511238585898485365, 0.9917933002572968393 ) ) ;
#6008=ADVANCED_FACE ( 'NONE', ( #30655 ), #6458, .F. ) ;
#6059=CARTESIAN_POINT ( 'NONE',  ( -60.64877780295373100, -2.458847256512897150, -1.115342769719651850 ) ) ;
#6091=CIRCLE ( 'NONE', #17719, 0.05000000000000009298 ) ;
#6092=EDGE_LOOP ( 'NONE', ( #4685, #7677, #7826, #8956, #27920, #26381 ) ) ;
#6103=EDGE_CURVE ( 'NONE', #7506, #4534, #15536, .T. ) ;
#6106=LINE ( 'NONE', #6252, #11653 ) ;
#6137=EDGE_CURVE ( 'NONE', #22178, #12162, #16597, .T. ) ;
#6154=B_SPLINE_CURVE_WITH_KNOTS ( 'NONE', 3,
 ( #22881, #29507, #5466, #3237, #7821, #10679, #24774, #3083, #17497, #12731, #20363, #27309, #12879 ),
 .UNSPECIFIED., .F., .F.,
 ( 4, 3, 3, 3, 4 ),
 ( 0.000000000000000000, 1.691191182548890470E-05, 3.382457420317648886E-05, 5.072228820803683589E-05, 6.090521770676877105E-05 ),
 .UNSPECIFIED. ) ;
#6173=AXIS2_PLACEMENT_3D ( 'NONE', #10920, #22828, #20301 ) ;
#6185=ADVANCED_FACE ( 'NONE', ( #2484 ), #29216, .F. ) ;
#6243=CARTESIAN_POINT ( 'NONE',  ( -73.89999999999997726, -2.435524336289708093E-15, 4.607889071584891164E-15 ) ) ;
#6252=CARTESIAN_POINT ( 'NONE',  ( -62.06710100716625789, -2.641521085243120570, -0.3278585316293294305 ) ) ;
#6257=CARTESIAN_POINT ( 'NONE',  ( -73.89999999999996305, 1.301636140808604125, 0.03242509391110788564 ) ) ;
#6259=DIRECTION ( 'NONE',  ( 0.000000000000000000, -0.9996898646859344595, -0.02490330187381124133 ) ) ;
#6272=VERTEX_POINT ( 'NONE', #26386 ) ;
#6301=CIRCLE ( 'NONE', #5282, 0.7500000000000002220 ) ;
#6316=DIRECTION ( 'NONE',  ( -1.000000000000000000, -3.053848253006669023E-16, 2.042510438544995169E-16 ) ) ;
#6327=ADVANCED_FACE ( 'NONE', ( #1180 ), #11019, .F. ) ;
#6381=LINE ( 'NONE', #28060, #9851 ) ;
#6384=DIRECTION ( 'NONE',  ( -3.002035892788116966E-16, 0.9996898646859343485, 0.02490330187381123786 ) ) ;
#6385=CARTESIAN_POINT ( 'NONE',  ( -61.34999999999997300, -2.574153985709302539, -0.5872647410103332133 ) ) ;
#6388=EDGE_CURVE ( 'NONE', #1635, #24203, #1492, .T. ) ;
#6393=VERTEX_POINT ( 'NONE', #25085 ) ;
#6399=ORIENTED_EDGE ( 'NONE', *, *, #20748, .T. ) ;
#6407=CARTESIAN_POINT ( 'NONE',  ( -61.34999999999997300, -2.551764585593653489, 0.6636807913650824009 ) ) ;
#6408=ORIENTED_EDGE ( 'NONE', *, *, #8812, .F. ) ;
#6414=ORIENTED_EDGE ( 'NONE', *, *, #21399, .F. ) ;
#6458=TOROIDAL_SURFACE ( 'NONE', #24160, 2.750000000000000444, 0.05000000000000000278 ) ;
#6474=ORIENTED_EDGE ( 'NONE', *, *, #20748, .F. ) ;
#6492=CARTESIAN_POINT ( 'NONE',  ( -62.09999999999998010, -2.687391533643786801, 0.2606275981160442456 ) ) ;
#6494=DIRECTION ( 'NONE',  ( 0.000000000000000000, 0.9996898646859345705, 0.02490330187381124133 ) ) ;
#6520=ORIENTED_EDGE ( 'NONE', *, *, #16270, .F. ) ;
#6548=EDGE_CURVE ( 'NONE', #19690, #21812, #16165, .T. ) ;
#6554=AXIS2_PLACEMENT_3D ( 'NONE', #28478, #26097, #24040 ) ;
#6575=CARTESIAN_POINT ( 'NONE',  ( -64.28602961791190751, -2.263268244922574279, -0.05638033785850377760 ) ) ;
#6587=CARTESIAN_POINT ( 'NONE',  ( -73.90999999999998238, -2.438578184542714499E-15, 4.609931582023435380E-15 ) ) ;
#6603=CARTESIAN_POINT ( 'NONE',  ( -62.39999999999998437, 1.076401154667962023E-15, 2.259002067258145746E-15 ) ) ;
#6682=EDGE_CURVE ( 'NONE', #3316, #29446, #28309, .T. ) ;
#6715=CARTESIAN_POINT ( 'NONE',  ( -62.04999999999998295, 2.699162634652024106, 0.06723891505929237289 ) ) ;
#6718=CARTESIAN_POINT ( 'NONE',  ( -60.59999999999997300, 1.626093840209163176E-15, 1.891350188320046374E-15 ) ) ;
#6783=EDGE_CURVE ( 'NONE', #7611, #24164, #23772, .T. ) ;
#6798=ORIENTED_EDGE ( 'NONE', *, *, #26658, .T. ) ;
#6811=CARTESIAN_POINT ( 'NONE',  ( -63.84999999999997300, -2.699162634652022774, -0.06723891505928747403 ) ) ;
#6826=CIRCLE ( 'NONE', #8335, 0.4600000000000000755 ) ;
#6828=ORIENTED_EDGE ( 'NONE', *, *, #15834, .F. ) ;
#6833=ORIENTED_EDGE ( 'NONE', *, *, #10888, .T. ) ;
#6835=CIRCLE ( 'NONE', #30073, 1.599188152294417131 ) ;
#6838=ORIENTED_EDGE ( 'NONE', *, *, #23497, .F. ) ;
#6880=ORIENTED_EDGE ( 'NONE', *, *, #7097, .F. ) ;
#6883=ADVANCED_FACE ( 'NONE', ( #31137 ), #9096, .F. ) ;
#6886=CARTESIAN_POINT ( 'NONE',  ( -62.09999999999997300, -2.736522795516423301, 0.2343065891546179669 ) ) ;
#6918=ORIENTED_EDGE ( 'NONE', *, *, #5083, .F. ) ;
#6940=CARTESIAN_POINT ( 'NONE',  ( -60.59999999999997300, -2.426837276046140079, -1.064406330116907329 ) ) ;
#6950=VERTEX_POINT ( 'NONE', #5633 ) ;
#6953=ORIENTED_EDGE ( 'NONE', *, *, #4164, .F. ) ;
#6961=LINE ( 'NONE', #18840, #30824 ) ;
#6963=DIRECTION ( 'NONE',  ( -1.000000000000000000, -3.053848253006669023E-16, 2.042510438544995415E-16 ) ) ;
#6964=CARTESIAN_POINT ( 'NONE',  ( -64.31974649313019654, 4.901397072418226544E-16, 2.651112292416007398E-15 ) ) ;
#6977=FACE_OUTER_BOUND ( 'NONE', #13420, .T. ) ;
#7019=CARTESIAN_POINT ( 'NONE',  ( -60.87073935753598164, -2.495861326358214782, -1.035156648315508354 ) ) ;
#7027=ORIENTED_EDGE ( 'NONE', *, *, #14666, .T. ) ;
#7053=ORIENTED_EDGE ( 'NONE', *, *, #10648, .F. ) ;
#7055=CARTESIAN_POINT ( 'NONE',  ( -62.09999999999997300, -2.712337243103304374, 0.1831892273270349092 ) ) ;
#7079=VERTEX_POINT ( 'NONE', #418 ) ;
#7093=AXIS2_PLACEMENT_3D ( 'NONE', #10837, #27464, #707 ) ;
#7097=EDGE_CURVE ( 'NONE', #26416, #10954, #13178, .T. ) ;
#7112=PRODUCT_DEFINITION_SHAPE ( 'NONE', 'NONE',  #15141 ) ;
#7113=ORIENTED_EDGE ( 'NONE', *, *, #7190, .T. ) ;
#7118=CARTESIAN_POINT ( 'NONE',  ( -62.09999999999997300, 1.168016602258162478E-15, 2.197726754101795588E-15 ) ) ;
#7134=CARTESIAN_POINT ( 'NONE',  ( -73.89999999999997726, -2.435524336289708093E-15, 4.607889071584891164E-15 ) ) ;
#7136=VECTOR ( 'NONE', #74, 1000.000000000000000 ) ;
#7137=CARTESIAN_POINT ( 'NONE',  ( -62.06730027881287981, -2.642931028823815254, 0.1961448473822917093 ) ) ;
#7161=EDGE_CURVE ( 'NONE', #5085, #16145, #6091, .T. ) ;
#7165=EDGE_CURVE ( 'NONE', #6950, #6393, #6106, .T. ) ;
#7190=EDGE_CURVE ( 'NONE', #21138, #31077, #16193, .T. ) ;
#7204=CARTESIAN_POINT ( 'NONE',  ( -62.09999999999997300, -2.687645153391445163, 0.1623166891292948111 ) ) ;
#7215=ORIENTED_EDGE ( 'NONE', *, *, #12507, .F. ) ;
#7267=CARTESIAN_POINT ( 'NONE',  ( -61.34999999999997300, -2.588576612942594668, -0.5896429294185620007 ) ) ;
#7274=( BOUNDED_SURFACE ( )  B_SPLINE_SURFACE ( 3, 2, ( 
 ( #30870, #28177, #14079 ),
 ( #11564, #1898, #19007 ),
 ( #30714, #11862, #25953 ),
 ( #1570, #6492, #14234 ) ),
 .UNSPECIFIED., .F., .F., .F. ) 
 B_SPLINE_SURFACE_WITH_KNOTS ( ( 4, 4 ),
 ( 3, 3 ),
 ( 6.485788022086533158E-05, 0.0002376820751398764635 ),
 ( 0.000000000000000000, 1.000000000000000000 ),
 .UNSPECIFIED. ) 
 GEOMETRIC_REPRESENTATION_ITEM ( )  RATIONAL_B_SPLINE_SURFACE ( (
 ( 1.000000000000000000, 0.8191520442890480869, 1.000000000000000000),
 ( 1.000000000000000000, 0.8271241339490560396, 1.000000000000000000),
 ( 1.000000000000000000, 0.7737134445967045471, 1.000000000000000000),
 ( 1.000000000000000000, 0.7071067811865996422, 1.000000000000000000) ) ) 
 REPRESENTATION_ITEM ( '' )  SURFACE ( )  );
#7277=CARTESIAN_POINT ( 'NONE',  ( -62.05843735016853202, -2.684085269283162045, 0.2308628115494030242 ) ) ;
#7281=ADVANCED_FACE ( 'NONE', ( #28567 ), #16379, .T. ) ;
#7285=ORIENTED_EDGE ( 'NONE', *, *, #14514, .T. ) ;
#7294=ORIENTED_EDGE ( 'NONE', *, *, #26442, .F. ) ;
#7321=CIRCLE ( 'NONE', #4282, 0.04999999999999988481 ) ;
#7326=CARTESIAN_POINT ( 'NONE',  ( -44.49999999999997868, 2.624185894800584062, 0.06537116741875480252 ) ) ;
#7328=CIRCLE ( 'NONE', #8816, 0.04999999999999988481 ) ;
#7366=AXIS2_PLACEMENT_3D ( 'NONE', #24727, #3041, #22690 ) ;
#7393=AXIS2_PLACEMENT_3D ( 'NONE', #13325, #30127, #10525 ) ;
#7399=EDGE_CURVE ( 'NONE', #21138, #3014, #4178, .T. ) ;
#7412=CONICAL_SURFACE ( 'NONE', #22667, 2.250000000000000444, 0.7853981633974536081 ) ;
#7418=VECTOR ( 'NONE', #28676, 1000.000000000000000 ) ;
#7428=DIRECTION ( 'NONE',  ( 3.002035892788117459E-16, -0.9996898646859344595, -0.02490330187381124133 ) ) ;
#7483=CARTESIAN_POINT ( 'NONE',  ( -61.36385676688671253, -2.559112712334371764, -0.8120304950550095713 ) ) ;
#7488=DIRECTION ( 'NONE',  ( 1.000000000000000000, 3.053848253006669023E-16, -2.042510438544995415E-16 ) ) ;
#7506=VERTEX_POINT ( 'NONE', #29201 ) ;
#7507=DIRECTION ( 'NONE',  ( 0.000000000000000000, -0.9996898646859343485, -0.02490330187381124133 ) ) ;
#7519=EDGE_CURVE ( 'NONE', #7079, #7997, #12394, .T. ) ;
#7523=FACE_OUTER_BOUND ( 'NONE', #14740, .T. ) ;
#7529=FACE_OUTER_BOUND ( 'NONE', #16183, .T. ) ;
#7539=PLANE ( 'NONE',  #27686 ) ;
#7546=ORIENTED_EDGE ( 'NONE', *, *, #2490, .F. ) ;
#7554=ADVANCED_FACE ( 'NONE', ( #19397 ), #3074, .F. ) ;
#7567=ORIENTED_EDGE ( 'NONE', *, *, #16202, .T. ) ;
#7577=AXIS2_PLACEMENT_3D ( 'NONE', #18021, #3606, #4071 ) ;
#7591=EDGE_LOOP ( 'NONE', ( #14875, #8237, #15722, #18107 ) ) ;
#7611=VERTEX_POINT ( 'NONE', #21070 ) ;
#7625=DIRECTION ( 'NONE',  ( -1.000000000000000000, -3.053848253006669023E-16, 2.042510438544995415E-16 ) ) ;
#7632=CARTESIAN_POINT ( 'NONE',  ( -61.37141394935931515, -2.563724941572514737, -0.8190313348002082883 ) ) ;
#7636=CARTESIAN_POINT ( 'NONE',  ( -62.09999999999997300, -2.673664601801277296, -0.2941788001767337013 ) ) ;
#7638=DIRECTION ( 'NONE',  ( 0.000000000000000000, 0.9996898646859339044, 0.02490330187382721813 ) ) ;
#7655=CYLINDRICAL_SURFACE ( 'NONE', #16122, 0.7500000000000002220 ) ;
#7658=CARTESIAN_POINT ( 'NONE',  ( -61.39999999999998437, -2.565822298769830478, -0.8405688140393350327 ) ) ;
#7659=ORIENTED_EDGE ( 'NONE', *, *, #15805, .F. ) ;
#7677=ORIENTED_EDGE ( 'NONE', *, *, #3780, .T. ) ;
#7685=VERTEX_POINT ( 'NONE', #4256 ) ;
#7705=CARTESIAN_POINT ( 'NONE',  ( -62.14999999999998437, 1.152747360993128871E-15, 2.207939306294521009E-15 ) ) ;
#7733=CARTESIAN_POINT ( 'NONE',  ( -62.06720320256510348, -2.648373711098206851, 0.1969833506954761504 ) ) ;
#7739=ADVANCED_FACE ( 'NONE', ( #14077 ), #19006, .F. ) ;
#7765=DIRECTION ( 'NONE',  ( 0.000000000000000000, -0.9996898646859344595, -0.02490330187381124133 ) ) ;
#7774=CARTESIAN_POINT ( 'NONE',  ( -62.09772439161942259, -2.519395624556878488, 0.1682286568119469583 ) ) ;
#7784=CARTESIAN_POINT ( 'NONE',  ( -61.39793805872155730, -2.653040316467372151, 0.5011856904451539307 ) ) ;
#7792=( NAMED_UNIT ( * ) SI_UNIT ( $, .STERADIAN. ) SOLID_ANGLE_UNIT ( ) );
#7806=LINE ( 'NONE', #17184, #19526 ) ;
#7821=CARTESIAN_POINT ( 'NONE',  ( -62.09529625801577168, -2.507189385900795653, -0.2994239205180544983 ) ) ;
#7823=FACE_BOUND ( 'NONE', #27826, .T. ) ;
#7824=CARTESIAN_POINT ( 'NONE',  ( -61.37035765953427102, -2.600782770733796934, 0.6894593850982138061 ) ) ;
#7826=ORIENTED_EDGE ( 'NONE', *, *, #851, .T. ) ;
#7830=DIRECTION ( 'NONE',  ( 0.000000000000000000, 0.9996898646859344595, 0.02490330187381124133 ) ) ;
#7832=ORIENTED_EDGE ( 'NONE', *, *, #28716, .F. ) ;
#7876=CARTESIAN_POINT ( 'NONE',  ( -64.29999999999996874, 2.249302195543353200, 0.05603242921607794191 ) ) ;
#7882=CARTESIAN_POINT ( 'NONE',  ( -62.09999999999997300, -2.737158043526071172, 0.2654540351181889912 ) ) ;
#7883=TOROIDAL_SURFACE ( 'NONE', #19027, 2.750000000000000000, 0.05000000000000000278 ) ;
#7887=AXIS2_PLACEMENT_3D ( 'NONE', #20156, #29785, #25491 ) ;
#7891=CARTESIAN_POINT ( 'NONE',  ( -60.61073679674431958, -2.503406555032712699, 0.9604922998729967798 ) ) ;
#7904=UNCERTAINTY_MEASURE_WITH_UNIT (LENGTH_MEASURE( 1.000000000000000082E-05 ), #13777, 'distance_accuracy_value', 'NONE');
#7910=EDGE_LOOP ( 'NONE', ( #27271, #19846, #10796, #18255 ) ) ;
#7926=EDGE_CURVE ( 'NONE', #1734, #30371, #604, .T. ) ;
#7930=EDGE_CURVE ( 'NONE', #6393, #1641, #12345, .T. ) ;
#7936=DIRECTION ( 'NONE',  ( 1.000000000000000000, 3.053848253006669023E-16, -2.042510438544995415E-16 ) ) ;
#7975=AXIS2_PLACEMENT_3D ( 'NONE', #28651, #29111, #7428 ) ;
#7997=VERTEX_POINT ( 'NONE', #10730 ) ;
#8002=CARTESIAN_POINT ( 'NONE',  ( -61.09509470490392147, -2.525749930366390394, 0.7571355657749674339 ) ) ;
#8025=DIRECTION ( 'NONE',  ( 0.000000000000000000, -0.9996898646859344595, -0.02490330187381124827 ) ) ;
#8038=ORIENTED_EDGE ( 'NONE', *, *, #10025, .T. ) ;
#8047=LINE ( 'NONE', #7876, #16572 ) ;
#8061=CARTESIAN_POINT ( 'NONE',  ( -60.60807700862574166, -2.500243950683068928, 0.9573076586908287888 ) ) ;
#8063=DIRECTION ( 'NONE',  ( 0.000000000000000000, -0.9996898646859344595, -0.02490330187381124480 ) ) ;
#8071=ORIENTED_EDGE ( 'NONE', *, *, #20534, .T. ) ;
#8081=ORIENTED_EDGE ( 'NONE', *, *, #19438, .F. ) ;
#8099=CARTESIAN_POINT ( 'NONE',  ( -62.10000000000010090, -2.520192335802873274, 0.1557817865423931636 ) ) ;
#8105=DIRECTION ( 'NONE',  ( 0.000000000000000000, 0.9996898646859343485, 0.02490330187381124133 ) ) ;
#8111=CARTESIAN_POINT ( 'NONE',  ( -61.39919398045554289, -2.652907018884305135, 0.5020538984275566552 ) ) ;
#8115=EDGE_CURVE ( 'NONE', #14916, #30026, #17800, .T. ) ;
#8130=DIRECTION ( 'NONE',  ( 1.000000000000000000, 3.053848253006669023E-16, -2.042510438544995415E-16 ) ) ;
#8138=CARTESIAN_POINT ( 'NONE',  ( -60.84461143194912580, -2.378894296791489449, 0.8519906293918184659 ) ) ;
#8163=CARTESIAN_POINT ( 'NONE',  ( -61.34999999999997300, -2.560800045841856942, 0.6641068371778564572 ) ) ;
#8210=CARTESIAN_POINT ( 'NONE',  ( -60.64271989919365780, -2.512715456726746677, 0.9876222387486196519 ) ) ;
#8215=ORIENTED_EDGE ( 'NONE', *, *, #28349, .F. ) ;
#8237=ORIENTED_EDGE ( 'NONE', *, *, #10400, .T. ) ;
#8246=AXIS2_PLACEMENT_3D ( 'NONE', #5029, #24202, #2510 ) ;
#8247=CARTESIAN_POINT ( 'NONE',  ( -62.09999999999997300, -2.520404473256288469, 0.1522704540930145123 ) ) ;
#8278=CARTESIAN_POINT ( 'NONE',  ( -61.34999999999997300, -2.515554072771550853, -0.7899129066418597578 ) ) ;
#8279=CARTESIAN_POINT ( 'NONE',  ( -74.38999999999998636, -2.585162900687033808E-15, 4.707972083073595634E-15 ) ) ;
#8282=ADVANCED_FACE ( 'NONE', ( #31300 ), #28616, .T. ) ;
#8286=DIRECTION ( 'NONE',  ( -1.000000000000000000, -3.053848253006669023E-16, 2.042510438544995415E-16 ) ) ;
#8297=FACE_OUTER_BOUND ( 'NONE', #11888, .T. ) ;
#8335=AXIS2_PLACEMENT_3D ( 'NONE', #27276, #25038, #7507 ) ;
#8340=DIRECTION ( 'NONE',  ( 1.000000000000000000, 3.053848253006669023E-16, -2.042510438544995415E-16 ) ) ;
#8360=CARTESIAN_POINT ( 'NONE',  ( -64.29999999999996874, -2.249302195543352312, -0.05603242921607237692 ) ) ;
#8384=AXIS2_PLACEMENT_3D ( 'NONE', #17030, #26509, #12714 ) ;
#8396=VECTOR ( 'NONE', #193, 1000.000000000000227 ) ;
#8405=EDGE_LOOP ( 'NONE', ( #29740, #28881, #18292, #20486 ) ) ;
#8433=CIRCLE ( 'NONE', #5915, 0.01000000000000001929 ) ;
#8444=DIRECTION ( 'NONE',  ( 0.000000000000000000, 0.9996898646859343485, 0.02490330187381130031 ) ) ;
#8447=CYLINDRICAL_SURFACE ( 'NONE', #8893, 2.700000000000000178 ) ;
#8454=EDGE_LOOP ( 'NONE', ( #18990, #20551, #2866, #434 ) ) ;
#8461=TOROIDAL_SURFACE ( 'NONE', #26163, 2.750000000000000000, 0.05000000000000000278 ) ;
#8467=ADVANCED_FACE ( 'NONE', ( #23362 ), #22863, .T. ) ;
#8474=EDGE_CURVE ( 'NONE', #8800, #20516, #16783, .T. ) ;
#8479=EDGE_CURVE ( 'NONE', #26621, #20326, #14231, .T. ) ;
#8537=CIRCLE ( 'NONE', #10560, 1.351996603031850208 ) ;
#8573=ORIENTED_EDGE ( 'NONE', *, *, #22922, .T. ) ;
#8577=SURFACE_SIDE_STYLE ('',( #4140 ) ) ;
#8581=AXIS2_PLACEMENT_3D ( 'NONE', #22351, #10301, #7765 ) ;
#8592=CARTESIAN_POINT ( 'NONE',  ( -60.64999999999998437, 2.699162634652024551, 0.06723891505929238677 ) ) ;
#8596=DIRECTION ( 'NONE',  ( -2.117927888850090838E-16, 0.02490330187381123786, -0.9996898646859343485 ) ) ;
#8603=FACE_OUTER_BOUND ( 'NONE', #15956, .T. ) ;
#8614=ORIENTED_EDGE ( 'NONE', *, *, #31068, .T. ) ;
#8620=CARTESIAN_POINT ( 'NONE',  ( -61.58692253671846828, -2.617039774925715268, 0.3716872663236084340 ) ) ;
#8625=CARTESIAN_POINT ( 'NONE',  ( -62.09999999999997300, -2.738044307818161549, 0.2465463003561280952 ) ) ;
#8631=CARTESIAN_POINT ( 'NONE',  ( -61.10430241999939938, -2.596047117859637154, 0.7520320166841959475 ) ) ;
#8636=DIRECTION ( 'NONE',  ( 0.000000000000000000, -0.9996898646859344595, -0.02490330187381124480 ) ) ;
#8674=ORIENTED_EDGE ( 'NONE', *, *, #2101, .F. ) ;
#8675=CARTESIAN_POINT ( 'NONE',  ( -73.89999999999997726, 0.7497673985144486242, 0.01867747640536001827 ) ) ;
#8701=ADVANCED_FACE ( 'NONE', ( #23506 ), #1803, .T. ) ;
#8712=ORIENTED_EDGE ( 'NONE', *, *, #19425, .T. ) ;
#8726=ORIENTED_EDGE ( 'NONE', *, *, #25114, .T. ) ;
#8742=ORIENTED_EDGE ( 'NONE', *, *, #16715, .F. ) ;
#8762=B_SPLINE_CURVE_WITH_KNOTS ( 'NONE', 3,
 ( #12826, #20155, #22508, #27255, #15541, #19830, #503, #29459, #7774, #10309, #29784, #8099, #8247 ),
 .UNSPECIFIED., .F., .F.,
 ( 4, 3, 3, 3, 4 ),
 ( 8.131516293641283255E-20, 1.679636492926620125E-05, 3.358850293755425803E-05, 5.044195101993695514E-05, 6.090334109303062704E-05 ),
 .UNSPECIFIED. ) ;
#8769=CARTESIAN_POINT ( 'NONE',  ( -73.89999999999997726, -2.435524336289708093E-15, 4.607889071584891164E-15 ) ) ;
#8774=CARTESIAN_POINT ( 'NONE',  ( -61.11832338958137711, -2.528658595614148741, 0.7486059352628685604 ) ) ;
#8783=ORIENTED_EDGE ( 'NONE', *, *, #12718, .F. ) ;
#8790=CARTESIAN_POINT ( 'NONE',  ( -62.29999999999998295, 2.749147127886321318, 0.06848408015298348972 ) ) ;
#8794=DIRECTION ( 'NONE',  ( -1.000000000000000000, -3.053848253006669023E-16, 2.042510438544995415E-16 ) ) ;
#8797=DIRECTION ( 'NONE',  ( 1.000000000000000000, 3.053848253006669023E-16, -2.042510438544995415E-16 ) ) ;
#8800=VERTEX_POINT ( 'NONE', #24441 ) ;
#8812=EDGE_CURVE ( 'NONE', #18413, #21138, #27404, .T. ) ;
#8816=AXIS2_PLACEMENT_3D ( 'NONE', #25757, #18485, #13236 ) ;
#8824=CIRCLE ( 'NONE', #26542, 2.700000000000000178 ) ;
#8829=VERTEX_POINT ( 'NONE', #10765 ) ;
#8832=DIRECTION ( 'NONE',  ( 1.000000000000000000, 3.053848253006669023E-16, -2.042510438544995169E-16 ) ) ;
#8849=CARTESIAN_POINT ( 'NONE',  ( -62.04999999999998295, -2.671081280896084653, -0.3941126626315437642 ) ) ;
#8854=CARTESIAN_POINT ( 'NONE',  ( -67.34999999999998010, -2.149333209074760109, -0.05354209902869064286 ) ) ;
#8858=CARTESIAN_POINT ( 'NONE',  ( -64.29999999999996874, 4.961699865966959239E-16, 2.647079050581693988E-15 ) ) ;
#8893=AXIS2_PLACEMENT_3D ( 'NONE', #18129, #11444, #1309 ) ;
#8896=CIRCLE ( 'NONE', #26611, 2.800000000000000266 ) ;
#8914=DIRECTION ( 'NONE',  ( -3.002035892788116966E-16, 0.9996898646859343485, 0.02490330187381124133 ) ) ;
#8915=DIRECTION ( 'NONE',  ( 3.002035892788117952E-16, -0.9996898646859344595, -0.02490330187381124133 ) ) ;
#8931=FACE_BOUND ( 'NONE', #10499, .T. ) ;
#8933=EDGE_LOOP ( 'NONE', ( #8742, #26296 ) ) ;
#8937=CIRCLE ( 'NONE', #18073, 0.7500000000000002220 ) ;
#8956=ORIENTED_EDGE ( 'NONE', *, *, #2074, .T. ) ;
#8964=CONICAL_SURFACE ( 'NONE', #24649, 1.350000000000000089, 0.04164257909858841422 ) ;
#8969=ADVANCED_FACE ( 'NONE', ( #6977 ), #21595, .T. ) ;
#8983=CARTESIAN_POINT ( 'NONE',  ( -61.34999999999997300, 1.397055221233662433E-15, 2.044538471210920981E-15 ) ) ;
#8984=AXIS2_PLACEMENT_3D ( 'NONE', #4669, #14324, #24450 ) ;
#8994=CARTESIAN_POINT ( 'NONE',  ( -74.39999999999997726, -2.588216748940040213E-15, 4.710014593512140639E-15 ) ) ;
#8995=ORIENTED_EDGE ( 'NONE', *, *, #22498, .F. ) ;
#9010=DIRECTION ( 'NONE',  ( 0.000000000000000000, -0.9996898646859344595, -0.02490330187381124133 ) ) ;
#9018=AXIS2_PLACEMENT_3D ( 'NONE', #25987, #9060, #11596 ) ;
#9023=B_SPLINE_CURVE_WITH_KNOTS ( 'NONE', 3,
 ( #12369, #17295, #19689, #5414, #29324, #7636, #18088, #20774, #28025, #15544, #22688, #20158, #1432, #3803, #13447, #25348 ),
 .UNSPECIFIED., .F., .F.,
 ( 4, 3, 3, 3, 3, 4 ),
 ( 0.000000000000000000, 2.715478742569115014E-05, 6.149153169279458048E-05, 9.810361480504433687E-05, 0.0001359429311246336211, 0.0001737107874904862475 ),
 .UNSPECIFIED. ) ;
#9034=CARTESIAN_POINT ( 'NONE',  ( -62.09999999999998010, -2.684508219953025243, -0.3645818587800867538 ) ) ;
#9060=DIRECTION ( 'NONE',  ( 0.000000000000000000, 0.000000000000000000, 1.000000000000000000 ) ) ;
#9068=DIRECTION ( 'NONE',  ( 0.000000000000000000, -0.9996898646859343485, -0.02490330187381123786 ) ) ;
#9070=( LENGTH_UNIT ( ) NAMED_UNIT ( * ) SI_UNIT ( .MILLI., .METRE. ) );
#9076=FACE_OUTER_BOUND ( 'NONE', #6092, .T. ) ;
#9096=TOROIDAL_SURFACE ( 'NONE', #18236, 2.750000000000000444, 0.05000000000000000278 ) ;
#9100=DIRECTION ( 'NONE',  ( 0.000000000000000000, 0.9996898646859343485, 0.02490330187381116153 ) ) ;
#9104=ORIENTED_EDGE ( 'NONE', *, *, #6682, .F. ) ;
#9127=ORIENTED_EDGE ( 'NONE', *, *, #16317, .T. ) ;
#9145=DIRECTION ( 'NONE',  ( -1.000000000000000000, -3.053848253006669023E-16, 2.042510438544995415E-16 ) ) ;
#9146=DIRECTION ( 'NONE',  ( -1.000000000000000000, -3.053848253006669023E-16, 2.042510438544995415E-16 ) ) ;
#9177=EDGE_CURVE ( 'NONE', #6393, #28678, #29679, .T. ) ;
#9179=CARTESIAN_POINT ( 'NONE',  ( -67.36397038208805554, 2.135367159695519934, 0.05319419038626561902 ) ) ;
#9181=ORIENTED_EDGE ( 'NONE', *, *, #5083, .T. ) ;
#9192=APPLICATION_CONTEXT ( 'automotive_design' ) ;
#9205=AXIS2_PLACEMENT_3D ( 'NONE', #5962, #1500, #15901 ) ;
#9217=CARTESIAN_POINT ( 'NONE',  ( -63.82928932188132620, 6.399178848011186396E-16, 2.550935903222500290E-15 ) ) ;
#9239=CARTESIAN_POINT ( 'NONE',  ( -61.09488783161975789, -2.368993871844102372, -0.8791439831129040927 ) ) ;
#9269=CARTESIAN_POINT ( 'NONE',  ( -62.09999999999997300, -2.667934001961814516, 0.1539767545844223928 ) ) ;
#9305=ADVANCED_FACE ( 'NONE', ( #7523 ), #5410, .T. ) ;
#9318=ORIENTED_EDGE ( 'NONE', *, *, #22937, .F. ) ;
#9353=CARTESIAN_POINT ( 'NONE',  ( -62.09999999999998010, -2.720545749060827134, -0.4014110452728690825 ) ) ;
#9458=VERTEX_POINT ( 'NONE', #8592 ) ;
#9461=CARTESIAN_POINT ( 'NONE',  ( -67.36397038208805554, -4.395200732636863594E-16, 3.272898199462452353E-15 ) ) ;
#9462=PLANE ( 'NONE',  #886 ) ;
#9463=ADVANCED_FACE ( 'NONE', ( #20494 ), #10478, .T. ) ;
#9467=AXIS2_PLACEMENT_3D ( 'NONE', #27879, #10778, #25493 ) ;
#9471=AXIS2_PLACEMENT_3D ( 'NONE', #11726, #3967, #13607 ) ;
#9474=CIRCLE ( 'NONE', #27645, 0.04999999999999988481 ) ;
#9528=CARTESIAN_POINT ( 'NONE',  ( -62.06710100716626499, -2.624587610216423172, -0.3274367013645040903 ) ) ;
#9530=LINE ( 'NONE', #6811, #7418 ) ;
#9571=CARTESIAN_POINT ( 'NONE',  ( -62.09999999999997300, 1.168016602258162478E-15, 2.197726754101795588E-15 ) ) ;
#9580=ORIENTED_EDGE ( 'NONE', *, *, #11524, .F. ) ;
#9585=CARTESIAN_POINT ( 'NONE',  ( -62.09999999999997300, 1.168016602258162478E-15, 2.197726754101795588E-15 ) ) ;
#9591=DIRECTION ( 'NONE',  ( 1.000000000000000000, 3.053848253006669023E-16, -2.042510438544995415E-16 ) ) ;
#9595=CARTESIAN_POINT ( 'NONE',  ( -62.09999999999997300, -2.696106776338097699, 0.1686925953295615732 ) ) ;
#9638=CARTESIAN_POINT ( 'NONE',  ( -44.49999999999997868, -0.7497673985144445163, -0.01867747640535983439 ) ) ;
#9640=ADVANCED_FACE ( 'NONE', ( #4774 ), #4504, .T. ) ;
#9643=CARTESIAN_POINT ( 'NONE',  ( -60.49999999999997868, 1.656632322739229403E-15, 1.870925083934595927E-15 ) ) ;
#9654=CARTESIAN_POINT ( 'NONE',  ( -61.34573544359366082, -2.573773108005611210, -0.5888079060821346244 ) ) ;
#9659=CARTESIAN_POINT ( 'NONE',  ( -61.39999999999998437, 1.381785979968628826E-15, 2.054751023403646402E-15 ) ) ;
#9675=CARTESIAN_POINT ( 'NONE',  ( -62.08893835062482935, -2.688756313659543817, 0.2461493159769948258 ) ) ;
#9681=DIRECTION ( 'NONE',  ( -1.000000000000000000, -3.053848253006669023E-16, 2.042510438544995415E-16 ) ) ;
#9687=ORIENTED_EDGE ( 'NONE', *, *, #26658, .F. ) ;
#9722=DIRECTION ( 'NONE',  ( 1.000000000000000000, 3.053848253006669023E-16, -2.042510438544995415E-16 ) ) ;
#9777=DIRECTION ( 'NONE',  ( 0.000000000000000000, -0.9996898646859344595, -0.02490330187381124480 ) ) ;
#9789=EDGE_CURVE ( 'NONE', #30371, #10647, #23646, .T. ) ;
#9795=ORIENTED_EDGE ( 'NONE', *, *, #1150, .T. ) ;
#9829=ORIENTED_EDGE ( 'NONE', *, *, #19425, .F. ) ;
#9835=ORIENTED_EDGE ( 'NONE', *, *, #20469, .F. ) ;
#9851=VECTOR ( 'NONE', #27599, 999.9999999999998863 ) ;
#9879=CARTESIAN_POINT ( 'NONE',  ( -64.32138495697122949, 4.896393452479652361E-16, 2.651446950365857792E-15 ) ) ;
#9896=ORIENTED_EDGE ( 'NONE', *, *, #25422, .F. ) ;
#9935=ORIENTED_EDGE ( 'NONE', *, *, #16589, .F. ) ;
#9942=ORIENTED_EDGE ( 'NONE', *, *, #24706, .F. ) ;
#9951=CARTESIAN_POINT ( 'NONE',  ( -67.33025350686975230, -4.292234512154642818E-16, 3.266011492503604425E-15 ) ) ;
#9962=ADVANCED_FACE ( 'NONE', ( #11858 ), #27095, .T. ) ;
#10014=EDGE_CURVE ( 'NONE', #7506, #19797, #15033, .T. ) ;
#10025=EDGE_CURVE ( 'NONE', #28152, #24203, #8047, .T. ) ;
#10033=EDGE_LOOP ( 'NONE', ( #1515, #8726, #16250, #2271, #6408, #15125, #21452, #29258, #16520 ) ) ;
#10037=DIRECTION ( 'NONE',  ( -2.117927888850090838E-16, 0.02490330187381123786, -0.9996898646859343485 ) ) ;
#10051=EDGE_CURVE ( 'NONE', #18759, #25939, #18085, .T. ) ;
#10053=ADVANCED_FACE ( 'NONE', ( #449 ), #8461, .T. ) ;
#10083=EDGE_CURVE ( 'NONE', #31077, #14916, #28357, .T. ) ;
#10095=EDGE_CURVE ( 'NONE', #20372, #28072, #23806, .T. ) ;
#10102=CARTESIAN_POINT ( 'NONE',  ( -62.08887962957128792, -2.673162175134213392, -0.3797419985091401440 ) ) ;
#10115=CARTESIAN_POINT ( 'NONE',  ( -61.61493949811855231, -2.643639042166195274, -0.5548158911668893412 ) ) ;
#10117=CARTESIAN_POINT ( 'NONE',  ( -61.34999999999997300, -2.574153985709302539, -0.5872647410103332133 ) ) ;
#10125=DIRECTION ( 'NONE',  ( 1.000000000000000000, 3.053848253006669023E-16, -2.042510438544995415E-16 ) ) ;
#10137=CARTESIAN_POINT ( 'NONE',  ( -67.33025350686975230, -4.292234512154642818E-16, 3.266011492503604425E-15 ) ) ;
#10171=CARTESIAN_POINT ( 'NONE',  ( -61.35985865640643055, -2.638419680335174267, 0.4713968906680494064 ) ) ;
#10172=ORIENTED_EDGE ( 'NONE', *, *, #24864, .F. ) ;
#10173=DIRECTION ( 'NONE',  ( 2.117927888850090591E-16, -0.02490330187381111643, 0.9996898646859343485 ) ) ;
#10203=EDGE_LOOP ( 'NONE', ( #5470, #17178, #15630, #4170 ) ) ;
#10248=CARTESIAN_POINT ( 'NONE',  ( -62.07177862240501298, -2.624829244341188250, -0.3257396798314975417 ) ) ;
#10278=CARTESIAN_POINT ( 'NONE',  ( -63.82928932188132620, -2.699162634652022330, -0.06723891505928762669 ) ) ;
#10287=DIRECTION ( 'NONE',  ( 3.002035892788116966E-16, -0.9996898646859343485, -0.02490330187381123786 ) ) ;
#10301=DIRECTION ( 'NONE',  ( -1.000000000000000000, -3.053848253006669023E-16, 2.042510438544995415E-16 ) ) ;
#10309=CARTESIAN_POINT ( 'NONE',  ( -62.09889467716561740, -2.519749790771223630, 0.1627451747621806999 ) ) ;
#10316=DIRECTION ( 'NONE',  ( 0.9396926207859097602, -0.008517430876162936787, 0.3419140708010978136 ) ) ;
#10321=CARTESIAN_POINT ( 'NONE',  ( -61.37466933804601865, -2.649564458509630072, 0.4839885628739446499 ) ) ;
#10326=ORIENTED_EDGE ( 'NONE', *, *, #16317, .F. ) ;
#10343=AXIS2_PLACEMENT_3D ( 'NONE', #16217, #23669, #8914 ) ;
#10344=DIRECTION ( 'NONE',  ( -3.002035892788117952E-16, 0.9996898646859344595, 0.02490330187381124133 ) ) ;
#10347=EDGE_CURVE ( 'NONE', #5910, #30896, #22908, .T. ) ;
#10362=ADVANCED_FACE ( 'NONE', ( #25194 ), #12445, .F. ) ;
#10400=EDGE_CURVE ( 'NONE', #10954, #4977, #27554, .T. ) ;
#10427=CARTESIAN_POINT ( 'NONE',  ( -61.82620411128902305, -2.492743192708819944, -0.4118588219422569252 ) ) ;
#10428=ADVANCED_BREP_SHAPE_REPRESENTATION ( '', ( #26054, #9018 ), #15625 ) ;
#10446=AXIS2_PLACEMENT_3D ( 'NONE', #3549, #8286, #1017 ) ;
#10478=CONICAL_SURFACE ( 'NONE', #28167, 1.350000000000000089, 0.04164257909858841422 ) ;
#10499=EDGE_LOOP ( 'NONE', ( #6520, #7215 ) ) ;
#10523=CARTESIAN_POINT ( 'NONE',  ( -64.32138495697122949, -2.298612619042724958, -0.05726080253994958458 ) ) ;
#10525=DIRECTION ( 'NONE',  ( 0.000000000000000000, 0.9996898646859343485, 0.02490330187381116153 ) ) ;
#10530=ORIENTED_EDGE ( 'NONE', *, *, #30919, .F. ) ;
#10536=CARTESIAN_POINT ( 'NONE',  ( -61.35320637528415944, -2.582160856334464683, 0.6721421056772638458 ) ) ;
#10556=ADVANCED_FACE ( 'NONE', ( #4737 ), #21909, .F. ) ;
#10560=AXIS2_PLACEMENT_3D ( 'NONE', #2834, #306, #12488 ) ;
#10569=FACE_OUTER_BOUND ( 'NONE', #30682, .T. ) ;
#10588=EDGE_CURVE ( 'NONE', #19797, #7506, #8896, .T. ) ;
#10593=CARTESIAN_POINT ( 'NONE',  ( -60.60075002049966031, -2.485844148457513114, 0.9463202019723547798 ) ) ;
#10624=CARTESIAN_POINT ( 'NONE',  ( -73.89999999999996305, -1.301636140808608788, -0.03242509391109851813 ) ) ;
#10647=VERTEX_POINT ( 'NONE', #5065 ) ;
#10648=EDGE_CURVE ( 'NONE', #5085, #20372, #8537, .T. ) ;
#10679=CARTESIAN_POINT ( 'NONE',  ( -62.09248695497047521, -2.506581153329065170, -0.3044590188957451149 ) ) ;
#10682=CARTESIAN_POINT ( 'NONE',  ( -61.34999999999997300, -2.569640616537276490, 0.6664830392735136000 ) ) ;
#10694=DIRECTION ( 'NONE',  ( 0.000000000000000000, -0.9996898646859344595, -0.02490330187381124480 ) ) ;
#10701=DIRECTION ( 'NONE',  ( -1.000000000000000000, -3.053848253006669023E-16, 2.042510438544995415E-16 ) ) ;
#10707=ORIENTED_EDGE ( 'NONE', *, *, #12781, .F. ) ;
#10713=CYLINDRICAL_SURFACE ( 'NONE', #3613, 2.800000000000000266 ) ;
#10730=CARTESIAN_POINT ( 'NONE',  ( -74.39999999999997726, 0.4598573377555272290, 0.01145551886195788488 ) ) ;
#10748=DIRECTION ( 'NONE',  ( -1.000000000000000000, -3.053848253006669023E-16, 2.042510438544995415E-16 ) ) ;
#10765=CARTESIAN_POINT ( 'NONE',  ( -62.09999999999997300, -2.509696570289218442, -0.2775754403374581791 ) ) ;
#10768=FACE_OUTER_BOUND ( 'NONE', #29088, .T. ) ;
#10778=DIRECTION ( 'NONE',  ( -1.000000000000000000, -3.053848253006669023E-16, 2.042510438544995415E-16 ) ) ;
#10780=CYLINDRICAL_SURFACE ( 'NONE', #7366, 2.700000000000000178 ) ;
#10796=ORIENTED_EDGE ( 'NONE', *, *, #27010, .T. ) ;
#10806=DIRECTION ( 'NONE',  ( -1.000000000000000000, -3.053848253006669023E-16, 2.042510438544995415E-16 ) ) ;
#10825=ORIENTED_EDGE ( 'NONE', *, *, #7930, .F. ) ;
#10837=CARTESIAN_POINT ( 'NONE',  ( -67.92156587216960872, -6.098012745906804249E-16, 3.386787660360170602E-15 ) ) ;
#10870=CARTESIAN_POINT ( 'NONE',  ( -74.38999999999998636, -2.585162900687033808E-15, 4.707972083073595634E-15 ) ) ;
#10876=EDGE_LOOP ( 'NONE', ( #18250, #4373, #29486, #28600 ) ) ;
#10885=CARTESIAN_POINT ( 'NONE',  ( -61.58695197172909985, -2.476857586476660433, -0.4985707676156266865 ) ) ;
#10888=EDGE_CURVE ( 'NONE', #2488, #12162, #17082, .T. ) ;
#10915=VECTOR ( 'NONE', #11605, 1000.000000000000000 ) ;
#10920=CARTESIAN_POINT ( 'NONE',  ( -60.59999999999997300, 1.626093840209163176E-15, 1.891350188320046374E-15 ) ) ;
#10935=DIRECTION ( 'NONE',  ( 1.000000000000000000, 3.053848253006669023E-16, -2.042510438544995415E-16 ) ) ;
#10943=CARTESIAN_POINT ( 'NONE',  ( -74.39999999999997726, -1.249612330857420961, -0.03112912734225919270 ) ) ;
#10954=VERTEX_POINT ( 'NONE', #15740 ) ;
#10962=CIRCLE ( 'NONE', #23611, 1.250000000000000222 ) ;
#10998=ORIENTED_EDGE ( 'NONE', *, *, #6388, .T. ) ;
#11007=PLANE ( 'NONE',  #17725 ) ;
#11019=TOROIDAL_SURFACE ( 'NONE', #7093, 1.649144805949033898, 0.05000000000000000278 ) ;
#11022=CARTESIAN_POINT ( 'NONE',  ( -61.13542439536123396, -2.577561284301780109, 0.8105868630520219886 ) ) ;
#11029=CIRCLE ( 'NONE', #25178, 0.04999999999999980849 ) ;
#11065=CARTESIAN_POINT ( 'NONE',  ( -61.34999999999997300, -2.435425537339440449, 0.6665789166144534539 ) ) ;
#11092=CARTESIAN_POINT ( 'NONE',  ( -60.84484350713348277, -2.449279924104672101, -0.9721809163073110716 ) ) ;
#11096=CARTESIAN_POINT ( 'NONE',  ( -62.06406286214753010, -2.657709275935192128, -0.3428149037536382671 ) ) ;
#11126=AXIS2_PLACEMENT_3D ( 'NONE', #6718, #1799, #11298 ) ;
#11151=EDGE_LOOP ( 'NONE', ( #17018, #12548 ) ) ;
#11191=FACE_OUTER_BOUND ( 'NONE', #16584, .T. ) ;
#11192=CARTESIAN_POINT ( 'NONE',  ( -67.92156587216960872, 1.648633347906700797, 0.04106915093618024315 ) ) ;
#11212=ORIENTED_EDGE ( 'NONE', *, *, #12849, .T. ) ;
#11220=CARTESIAN_POINT ( 'NONE',  ( -62.04999999999998295, 1.183285843523195887E-15, 2.187514201909070562E-15 ) ) ;
#11222=CARTESIAN_POINT ( 'NONE',  ( -67.88621053311027254, -5.990042905486032463E-16, 3.379566295451473069E-15 ) ) ;
#11235=CARTESIAN_POINT ( 'NONE',  ( -73.89999999999997726, -2.435524336289708093E-15, 4.607889071584891164E-15 ) ) ;
#11243=CARTESIAN_POINT ( 'NONE',  ( -62.06727109562227440, -2.629110561070149288, -0.3274874463776150102 ) ) ;
#11253=VERTEX_POINT ( 'NONE', #25354 ) ;
#11258=( NAMED_UNIT ( * ) SI_UNIT ( $, .STERADIAN. ) SOLID_ANGLE_UNIT ( ) );
#11273=FACE_OUTER_BOUND ( 'NONE', #28250, .T. ) ;
#11279=DIRECTION ( 'NONE',  ( 0.000000000000000000, 0.9996898646859345705, 0.02490330187381124133 ) ) ;
#11298=DIRECTION ( 'NONE',  ( 3.002035892788116966E-16, -0.9996898646859343485, -0.02490330187381123786 ) ) ;
#11301=CARTESIAN_POINT ( 'NONE',  ( -73.84999999999996589, -2.420255095024673698E-15, 4.597676519392165349E-15 ) ) ;
#11330=DIRECTION ( 'NONE',  ( -1.000000000000000000, -3.053848253006669023E-16, 2.042510438544995415E-16 ) ) ;
#11332=CIRCLE ( 'NONE', #26511, 2.650000000000000799 ) ;
#11384=CIRCLE ( 'NONE', #3302, 0.05000000000000009298 ) ;
#11418=VECTOR ( 'NONE', #26393, 999.9999999999998863 ) ;
#11429=ORIENTED_EDGE ( 'NONE', *, *, #27672, .T. ) ;
#11444=DIRECTION ( 'NONE',  ( 1.000000000000000000, 3.053848253006669023E-16, -2.042510438544995415E-16 ) ) ;
#11480=CARTESIAN_POINT ( 'NONE',  ( -60.49999999999997868, 1.656632322739229403E-15, 1.870925083934595927E-15 ) ) ;
#11484=AXIS2_PLACEMENT_3D ( 'NONE', #27707, #8832, #5858 ) ;
#11513=CARTESIAN_POINT ( 'NONE',  ( -44.49999999999997868, 6.542789527549899840E-15, -1.397091617737396343E-15 ) ) ;
#11524=EDGE_CURVE ( 'NONE', #20372, #5085, #20204, .T. ) ;
#11536=DIRECTION ( 'NONE',  ( -1.000000000000000000, -3.053848253006669023E-16, 2.042510438544995415E-16 ) ) ;
#11555=EDGE_LOOP ( 'NONE', ( #884, #27229, #10998, #22075 ) ) ;
#11564=CARTESIAN_POINT ( 'NONE',  ( -62.09999999999998010, -2.698422353084989123, 0.1478368950964479289 ) ) ;
#11571=DIRECTION ( 'NONE',  ( 2.117927888850091331E-16, -0.02490330187381135929, 0.9996898646859343485 ) ) ;
#11596=DIRECTION ( 'NONE',  ( 1.000000000000000000, 0.000000000000000000, 0.000000000000000000 ) ) ;
#11605=DIRECTION ( 'NONE',  ( 1.000000000000000000, 3.053848253006669023E-16, -2.042510438544995415E-16 ) ) ;
#11653=VECTOR ( 'NONE', #25405, 999.9999999999998863 ) ;
#11670=CARTESIAN_POINT ( 'NONE',  ( -62.29999999999998295, -2.749147127886318653, -0.06848408015297868801 ) ) ;
#11691=EDGE_LOOP ( 'NONE', ( #11429, #7294, #6828, #30178 ) ) ;
#11701=DIRECTION ( 'NONE',  ( 1.000000000000000000, 3.053848253006669023E-16, -2.042510438544995415E-16 ) ) ;
#11703=DIRECTION ( 'NONE',  ( 0.000000000000000000, 0.9996898646859343485, 0.02490330187381123439 ) ) ;
#11715=VERTEX_POINT ( 'NONE', #20282 ) ;
#11726=CARTESIAN_POINT ( 'NONE',  ( -64.28602961791190751, 5.004363292900432036E-16, 2.644225585457161048E-15 ) ) ;
#11757=CARTESIAN_POINT ( 'NONE',  ( -61.11832338958127053, -2.488248221111335923, -0.8735822397580453869 ) ) ;
#11772=CARTESIAN_POINT ( 'NONE',  ( -62.09999999999997300, 2.699162634652024551, 0.06723891505929256718 ) ) ;
#11785=AXIS2_PLACEMENT_3D ( 'NONE', #1325, #30300, #8915 ) ;
#11791=CARTESIAN_POINT ( 'NONE',  ( -62.09999999999997300, -2.657853763656952140, 0.1506955384656827324 ) ) ;
#11797=EDGE_CURVE ( 'NONE', #25939, #28152, #18211, .T. ) ;
#11805=AXIS2_PLACEMENT_3D ( 'NONE', #5536, #3478, #5844 ) ;
#11838=ORIENTED_EDGE ( 'NONE', *, *, #14924, .F. ) ;
#11845=ORIENTED_EDGE ( 'NONE', *, *, #10051, .T. ) ;
#11858=FACE_OUTER_BOUND ( 'NONE', #2905, .T. ) ;
#11860=CARTESIAN_POINT ( 'NONE',  ( -61.35074338551757478, -2.593275822190189039, -0.5912877971683896394 ) ) ;
#11862=CARTESIAN_POINT ( 'NONE',  ( -62.09999999999998010, -2.699336478251256111, 0.2304543901385250337 ) ) ;
#11870=AXIS2_PLACEMENT_3D ( 'NONE', #1069, #8340, #18013 ) ;
#11872=CARTESIAN_POINT ( 'NONE',  ( -74.38999999999998636, 1.239615432210556367, 0.03088009432353080660 ) ) ;
#11874=CARTESIAN_POINT ( 'NONE',  ( -61.84504909419678143, -2.680454941414578851, 0.3368274758861355966 ) ) ;
#11888=EDGE_LOOP ( 'NONE', ( #2672, #13049, #1845, #3462 ) ) ;
#11902=ADVANCED_FACE ( 'NONE', ( #5035 ), #30382, .T. ) ;
#11910=VECTOR ( 'NONE', #12534, 999.9999999999998863 ) ;
#11921=CARTESIAN_POINT ( 'NONE',  ( -60.59999999999997300, -2.476825173781434852, 0.9422510591782664591 ) ) ;
#11933=AXIS2_PLACEMENT_3D ( 'NONE', #25154, #22324, #8063 ) ;
#11939=ORIENTED_EDGE ( 'NONE', *, *, #13248, .T. ) ;
#11951=DIRECTION ( 'NONE',  ( 0.000000000000000000, -0.9996898646859343485, -0.02490330187381124133 ) ) ;
#11961=DIRECTION ( 'NONE',  ( 1.000000000000000000, 3.053848253006669023E-16, -2.042510438544995415E-16 ) ) ;
#11980=DIRECTION ( 'NONE',  ( -1.000000000000000000, -3.053848253006669023E-16, 2.042510438544995415E-16 ) ) ;
#12023=DIRECTION ( 'NONE',  ( 1.000000000000000000, 3.053848253006669023E-16, -2.042510438544995415E-16 ) ) ;
#12087=DIRECTION ( 'NONE',  ( -1.000000000000000000, -3.053848253006669023E-16, 2.042510438544995415E-16 ) ) ;
#12117=CIRCLE ( 'NONE', #28295, 2.700000000000000178 ) ;
#12134=EDGE_CURVE ( 'NONE', #19797, #7685, #22779, .T. ) ;
#12162=VERTEX_POINT ( 'NONE', #14336 ) ;
#12173=CARTESIAN_POINT ( 'NONE',  ( -44.49999999999997868, -0.7497673985144445163, -0.01867747640535983439 ) ) ;
#12186=AXIS2_PLACEMENT_3D ( 'NONE', #25177, #790, #25329 ) ;
#12191=CARTESIAN_POINT ( 'NONE',  ( -62.04999999999998295, -2.687391533643777919, 0.2606275981160458555 ) ) ;
#12205=EDGE_LOOP ( 'NONE', ( #19761, #10825, #29436, #1959, #15890 ) ) ;
#12207=DIRECTION ( 'NONE',  ( 1.000000000000000000, 3.053848253006669023E-16, -2.042510438544995415E-16 ) ) ;
#12226=CARTESIAN_POINT ( 'NONE',  ( -61.39919102937894735, -2.565992354215222981, -0.8400338161548545068 ) ) ;
#12251=DIRECTION ( 'NONE',  ( -1.000000000000000000, -3.053848253006669023E-16, 2.042510438544995415E-16 ) ) ;
#12263=CARTESIAN_POINT ( 'NONE',  ( -63.84999999999997300, 6.335931579819947332E-16, 2.555166080847169934E-15 ) ) ;
#12264=CARTESIAN_POINT ( 'NONE',  ( -62.14999999999998437, 2.799131621120617641, 0.06972924524667370449 ) ) ;
#12277=CARTESIAN_POINT ( 'NONE',  ( -73.90999999999998238, -2.438578184542714499E-15, 4.609931582023435380E-15 ) ) ;
#12288=AXIS2_PLACEMENT_3D ( 'NONE', #29582, #5686, #22808 ) ;
#12289=EDGE_CURVE ( 'NONE', #7611, #24092, #14277, .T. ) ;
#12334=PRODUCT_DEFINITION_CONTEXT ( 'detailed design', #9192, 'design' ) ;
#12345=( BOUNDED_CURVE ( )  B_SPLINE_CURVE ( 3, ( #29893, #15487, #3465, #24826 ),
 .UNSPECIFIED., .F., .T. ) 
 B_SPLINE_CURVE_WITH_KNOTS ( ( 4, 4 ),
 ( 4.829242994979814796, 4.929162845165778961 ),
 .UNSPECIFIED. ) 
 CURVE ( )  GEOMETRIC_REPRESENTATION_ITEM ( )  RATIONAL_B_SPLINE_CURVE ( ( 1.000000000000000000, 0.9991681750023542197, 0.9991681750023542197, 1.000000000000000000 ) ) 
 REPRESENTATION_ITEM ( '' )  );
#12347=EDGE_CURVE ( 'NONE', #2409, #24563, #19859, .T. ) ;
#12355=ORIENTED_EDGE ( 'NONE', *, *, #19010, .T. ) ;
#12363=CARTESIAN_POINT ( 'NONE',  ( -61.35802040574235861, -2.553010640673968989, -0.8058083345264630548 ) ) ;
#12369=CARTESIAN_POINT ( 'NONE',  ( -62.09999999999997300, -2.625757682666624238, -0.2804666419185134485 ) ) ;
#12384=EDGE_LOOP ( 'NONE', ( #9795, #15078, #24165, #25859, #7285, #9835 ) ) ;
#12394=LINE ( 'NONE', #19712, #7136 ) ;
#12402=DIRECTION ( 'NONE',  ( 1.000000000000000000, 3.053848253006669023E-16, -2.042510438544995415E-16 ) ) ;
#12410=DIRECTION ( 'NONE',  ( -1.000000000000000000, -3.053848253006669023E-16, 2.042510438544995415E-16 ) ) ;
#12413=AXIS2_PLACEMENT_3D ( 'NONE', #30076, #7936, #3646 ) ;
#12425=CIRCLE ( 'NONE', #30118, 2.650000000000000799 ) ;
#12439=EDGE_CURVE ( 'NONE', #4710, #30753, #8937, .T. ) ;
#12445=TOROIDAL_SURFACE ( 'NONE', #7887, 2.299325721147392088, 0.05000000000000000278 ) ;
#12446=VECTOR ( 'NONE', #9722, 1000.000000000000000 ) ;
#12462=AXIS2_PLACEMENT_3D ( 'NONE', #20592, #10748, #18358 ) ;
#12469=CARTESIAN_POINT ( 'NONE',  ( -64.31974649313019654, 4.901397072418226544E-16, 2.651112292416007398E-15 ) ) ;
#12488=DIRECTION ( 'NONE',  ( 0.000000000000000000, -0.9996898646859343485, -0.02490330187381124133 ) ) ;
#12500=ORIENTED_EDGE ( 'NONE', *, *, #14263, .F. ) ;
#12501=ORIENTED_EDGE ( 'NONE', *, *, #28716, .T. ) ;
#12507=EDGE_CURVE ( 'NONE', #7079, #25398, #22124, .T. ) ;
#12521=DIRECTION ( 'NONE',  ( 0.000000000000000000, -0.9996898646859344595, -0.02490330187381124133 ) ) ;
#12534=DIRECTION ( 'NONE',  ( -3.002035892788117459E-16, 0.9996898646859344595, 0.02490330187381124133 ) ) ;
#12541=CARTESIAN_POINT ( 'NONE',  ( -61.37927097740655569, -2.651043540278919419, 0.4875364716318860703 ) ) ;
#12548=ORIENTED_EDGE ( 'NONE', *, *, #12439, .F. ) ;
#12608=FACE_OUTER_BOUND ( 'NONE', #20543, .T. ) ;
#12614=CARTESIAN_POINT ( 'NONE',  ( -62.34999999999997300, 1.091670395932995432E-15, 2.248789515065420326E-15 ) ) ;
#12633=CARTESIAN_POINT ( 'NONE',  ( -63.86464466094066239, -2.684522515537854925, -0.06687421464704190743 ) ) ;
#12638=CARTESIAN_POINT ( 'NONE',  ( -62.06644497648784409, -2.658467779542562859, 0.2005540737866994272 ) ) ;
#12642=DIRECTION ( 'NONE',  ( 0.000000000000000000, -0.9996898646859344595, -0.02490330187381124827 ) ) ;
#12672=DIRECTION ( 'NONE',  ( 0.000000000000000000, -0.9996898646859343485, -0.02490330187381124133 ) ) ;
#12675=FACE_OUTER_BOUND ( 'NONE', #8405, .T. ) ;
#12695=DIRECTION ( 'NONE',  ( 3.002035892788117459E-16, -0.9996898646859343485, -0.02490330187381124480 ) ) ;
#12714=DIRECTION ( 'NONE',  ( 0.000000000000000000, -0.9996898646859344595, -0.02490330187381124480 ) ) ;
#12718=EDGE_CURVE ( 'NONE', #1734, #1808, #19598, .T. ) ;
#12720=ADVANCED_FACE ( 'NONE', ( #29919 ), #22959, .T. ) ;
#12722=CARTESIAN_POINT ( 'NONE',  ( -60.49999999999997868, -2.624185894800576513, -0.06537116741875401149 ) ) ;
#12731=CARTESIAN_POINT ( 'NONE',  ( -62.07633557594488849, -2.504645164848317673, -0.3199649952759585636 ) ) ;
#12781=EDGE_CURVE ( 'NONE', #25939, #18759, #21639, .T. ) ;
#12788=CARTESIAN_POINT ( 'NONE',  ( -60.63660384741033482, -2.513063517893788568, 0.9832629503941247018 ) ) ;
#12808=DIRECTION ( 'NONE',  ( 1.000000000000000000, 3.053848253006669023E-16, -2.042510438544995415E-16 ) ) ;
#12810=DIRECTION ( 'NONE',  ( 0.000000000000000000, -0.9996898646859344595, -0.02490330187381105745 ) ) ;
#12826=CARTESIAN_POINT ( 'NONE',  ( -62.06710100716625789, -2.517118187348250213, 0.1993515260053453086 ) ) ;
#12849=EDGE_CURVE ( 'NONE', #21812, #5852, #18565, .T. ) ;
#12858=ORIENTED_EDGE ( 'NONE', *, *, #30925, .F. ) ;
#12879=CARTESIAN_POINT ( 'NONE',  ( -62.06710100716626499, -2.504070139480777613, -0.3244344873171103316 ) ) ;
#12890=ORIENTED_EDGE ( 'NONE', *, *, #17953, .F. ) ;
#12895=EDGE_CURVE ( 'NONE', #30896, #28721, #27108, .T. ) ;
#12909=FACE_OUTER_BOUND ( 'NONE', #27353, .T. ) ;
#12932=DIRECTION ( 'NONE',  ( 1.000000000000000000, 3.053848253006669023E-16, -2.042510438544995415E-16 ) ) ;
#12936=DIRECTION ( 'NONE',  ( 0.000000000000000000, 0.9996898646859343485, 0.02490330187381123439 ) ) ;
#12941=CARTESIAN_POINT ( 'NONE',  ( -62.04999999999998295, -2.671081280896084653, -0.3941126626315437642 ) ) ;
#12946=AXIS2_PLACEMENT_3D ( 'NONE', #25852, #15734, #21132 ) ;
#12962=CIRCLE ( 'NONE', #9471, 2.263970382088065225 ) ;
#12970=ORIENTED_EDGE ( 'NONE', *, *, #14756, .F. ) ;
#12971=DIRECTION ( 'NONE',  ( -1.000000000000000000, -3.053848253006669023E-16, 2.042510438544995169E-16 ) ) ;
#12972=CARTESIAN_POINT ( 'NONE',  ( -63.84999999999997300, 6.335931579819947332E-16, 2.555166080847169934E-15 ) ) ;
#12995=TOROIDAL_SURFACE ( 'NONE', #4418, 2.649999999999999911, 0.05000000000000000278 ) ;
#13015=ORIENTED_EDGE ( 'NONE', *, *, #16984, .F. ) ;
#13017=ORIENTED_EDGE ( 'NONE', *, *, #15779, .T. ) ;
#13036=CIRCLE ( 'NONE', #30743, 2.136029617911934686 ) ;
#13049=ORIENTED_EDGE ( 'NONE', *, *, #4164, .T. ) ;
#13055=EDGE_LOOP ( 'NONE', ( #28941, #28328, #30780, #8573 ) ) ;
#13062=ORIENTED_EDGE ( 'NONE', *, *, #10014, .F. ) ;
#13067=EDGE_CURVE ( 'NONE', #2901, #1734, #28178, .T. ) ;
#13072=CARTESIAN_POINT ( 'NONE',  ( -60.59540624230464800, -2.457874471988325205, 0.9407545623323243511 ) ) ;
#13109=CARTESIAN_POINT ( 'NONE',  ( -60.63087243001902493, -2.512277203407240034, 0.9787440703680012621 ) ) ;
#13134=CARTESIAN_POINT ( 'NONE',  ( -61.39879105983193597, -2.624675223805974511, -0.6332464253769281015 ) ) ;
#13136=ADVANCED_FACE ( 'NONE', ( #3288 ), #8964, .T. ) ;
#13147=DIRECTION ( 'NONE',  ( -3.002035892788116966E-16, 0.9996898646859343485, 0.02490330187381124133 ) ) ;
#13161=CARTESIAN_POINT ( 'NONE',  ( -60.60558231549867969, -2.446663424644156315, -1.077479343426181124 ) ) ;
#13178=( BOUNDED_CURVE ( )  B_SPLINE_CURVE ( 3, ( #30459, #8620, #3574, #13522 ),
 .UNSPECIFIED., .F., .T. ) 
 B_SPLINE_CURVE_WITH_KNOTS ( ( 4, 4 ),
 ( 1.354022462013807049, 1.453942312199770548 ),
 .UNSPECIFIED. ) 
 CURVE ( )  GEOMETRIC_REPRESENTATION_ITEM ( )  RATIONAL_B_SPLINE_CURVE ( ( 1.000000000000000000, 0.9991681750023542197, 0.9991681750023542197, 1.000000000000000000 ) ) 
 REPRESENTATION_ITEM ( '' )  );
#13180=CARTESIAN_POINT ( 'NONE',  ( -61.34999999999997300, -2.520040662139441778, -0.7900246721901127422 ) ) ;
#13185=CIRCLE ( 'NONE', #55, 0.01000000000000001929 ) ;
#13200=CARTESIAN_POINT ( 'NONE',  ( -61.36301639239449912, -2.595653720285160837, 0.6828058785558981381 ) ) ;
#13207=AXIS2_PLACEMENT_3D ( 'NONE', #15615, #20986, #10694 ) ;
#13209=CARTESIAN_POINT ( 'NONE',  ( -60.59999999999998010, -2.408745774756101188, -1.060314564156378037 ) ) ;
#13212=ADVANCED_FACE ( 'NONE', ( #1677, #1843 ), #9462, .T. ) ;
#13236=DIRECTION ( 'NONE',  ( 0.000000000000000000, -0.9996898646859343485, -0.02490330187381116153 ) ) ;
#13238=EDGE_LOOP ( 'NONE', ( #253, #13062, #15634, #17459 ) ) ;
#13245=CARTESIAN_POINT ( 'NONE',  ( -60.59999999999997300, -2.524216908331983866, -0.06288083723137120884 ) ) ;
#13248=EDGE_CURVE ( 'NONE', #27015, #24287, #15047, .T. ) ;
#13267=DIRECTION ( 'NONE',  ( 0.9396926207859090940, -0.008517430876162981890, 0.3419140708010995899 ) ) ;
#13268=PLANE ( 'NONE',  #14641 ) ;
#13290=LINE ( 'NONE', #15701, #4382 ) ;
#13296=DIRECTION ( 'NONE',  ( 1.000000000000000000, 3.053848253006669023E-16, -2.042510438544995415E-16 ) ) ;
#13300=CARTESIAN_POINT ( 'NONE',  ( -60.61746561950877066, -2.456658750590456908, -1.090869315165489128 ) ) ;
#13319=CARTESIAN_POINT ( 'NONE',  ( -61.34999999999997300, -2.482504579955461477, 0.4612981795977083577 ) ) ;
#13325=CARTESIAN_POINT ( 'NONE',  ( -62.39999999999998437, -2.749147127886319542, -0.06848408015297867413 ) ) ;
#13331=ADVANCED_FACE ( 'NONE', ( #1310 ), #7412, .T. ) ;
#13346=ORIENTED_EDGE ( 'NONE', *, *, #24338, .F. ) ;
#13357=AXIS2_PLACEMENT_3D ( 'NONE', #4684, #22118, #15122 ) ;
#13369=EDGE_LOOP ( 'NONE', ( #14580, #9935, #28374, #17563, #24134, #29687 ) ) ;
#13382=DIRECTION ( 'NONE',  ( 0.000000000000000000, -0.9996898646859344595, -0.02490330187381124480 ) ) ;
#13383=VERTEX_POINT ( 'NONE', #27915 ) ;
#13397=CIRCLE ( 'NONE', #31129, 1.599188152294417131 ) ;
#13398=CARTESIAN_POINT ( 'NONE',  ( -60.64877780295373810, -2.511331634963794190, 0.9915305058630268231 ) ) ;
#13420=EDGE_LOOP ( 'NONE', ( #12501, #29911, #11845, #17862 ) ) ;
#13447=CARTESIAN_POINT ( 'NONE',  ( -62.09999999999997300, -2.722373408723269161, -0.3890241620917929133 ) ) ;
#13470=FILL_AREA_STYLE_COLOUR ( '', #22208 ) ;
#13490=EDGE_CURVE ( 'NONE', #5852, #3831, #29155, .T. ) ;
#13511=FACE_OUTER_BOUND ( 'NONE', #14478, .T. ) ;
#13516=VERTEX_POINT ( 'NONE', #30757 ) ;
#13522=CARTESIAN_POINT ( 'NONE',  ( -62.06710100716625789, -2.637635658083895329, 0.1963493119579511614 ) ) ;
#13560=DIRECTION ( 'NONE',  ( 2.117927888850091331E-16, -0.02490330187381135929, 0.9996898646859343485 ) ) ;
#13603=CARTESIAN_POINT ( 'NONE',  ( -61.34999999999997300, -2.661068980108069137, 0.4568499568858441773 ) ) ;
#13604=CARTESIAN_POINT ( 'NONE',  ( -61.39999999999998437, -2.652806974455509170, 0.5026083527760007996 ) ) ;
#13607=DIRECTION ( 'NONE',  ( 0.000000000000000000, 0.9996898646859343485, 0.02490330187381124133 ) ) ;
#13611=CARTESIAN_POINT ( 'NONE',  ( -62.06125279754600399, -2.664633900085208396, -0.3536699491376213977 ) ) ;
#13620=CARTESIAN_POINT ( 'NONE',  ( -63.86464466094066239, 2.684522515537854481, 0.06687421464704730589 ) ) ;
#13638=EDGE_CURVE ( 'NONE', #12162, #22178, #18121, .T. ) ;
#13682=CARTESIAN_POINT ( 'NONE',  ( -67.88621053311027254, -1.613288973786559444, -0.04018868625472774014 ) ) ;
#13713=EDGE_CURVE ( 'NONE', #24203, #2488, #26623, .T. ) ;
#13751=CARTESIAN_POINT ( 'NONE',  ( -63.82928932188132620, 2.649178141417727339, 0.06599374996560235240 ) ) ;
#13762=FACE_OUTER_BOUND ( 'NONE', #20044, .T. ) ;
#13777=( LENGTH_UNIT ( ) NAMED_UNIT ( * ) SI_UNIT ( .MILLI., .METRE. ) );
#13797=DIRECTION ( 'NONE',  ( -1.000000000000000000, -3.053848253006669023E-16, 2.042510438544995415E-16 ) ) ;
#13814=ORIENTED_EDGE ( 'NONE', *, *, #7161, .F. ) ;
#13816=CARTESIAN_POINT ( 'NONE',  ( -60.59999999999997300, 2.524216908331987419, 0.06288083723137531666 ) ) ;
#13822=DIRECTION ( 'NONE',  ( -1.000000000000000000, -3.053848253006669023E-16, 2.042510438544995415E-16 ) ) ;
#13837=CONICAL_SURFACE ( 'NONE', #5777, 2.150000000000000355, 0.03277514440407566787 ) ;
#13839=EDGE_CURVE ( 'NONE', #30026, #6950, #24952, .T. ) ;
#13850=CARTESIAN_POINT ( 'NONE',  ( -74.39999999999997726, -2.588216748940040213E-15, 4.710014593512140639E-15 ) ) ;
#13851=ORIENTED_EDGE ( 'NONE', *, *, #1402, .F. ) ;
#13862=DIRECTION ( 'NONE',  ( -1.000000000000000000, -3.053848253006669023E-16, 2.042510438544995415E-16 ) ) ;
#13865=CARTESIAN_POINT ( 'NONE',  ( -62.09999999999997300, -2.524216908331983422, -0.06288083723137104231 ) ) ;
#13900=CARTESIAN_POINT ( 'NONE',  ( -61.37134253426428643, -2.620685193807273272, -0.6125669275117787693 ) ) ;
#13929=VERTEX_POINT ( 'NONE', #13865 ) ;
#13932=CIRCLE ( 'NONE', #8384, 2.625000000000000444 ) ;
#13937=EDGE_LOOP ( 'NONE', ( #13814, #9580, #6399, #17210 ) ) ;
#13954=VECTOR ( 'NONE', #23477, 1000.000000000000227 ) ;
#13956=SURFACE_SIDE_STYLE ('',( #30432 ) ) ;
#13968=CARTESIAN_POINT ( 'NONE',  ( -61.34999999999997300, -2.609922480197373940, 0.4591346723570145505 ) ) ;
#13979=EDGE_LOOP ( 'NONE', ( #25756, #24002 ) ) ;
#14068=VERTEX_POINT ( 'NONE', #9638 ) ;
#14077=FACE_OUTER_BOUND ( 'NONE', #3311, .T. ) ;
#14079=CARTESIAN_POINT ( 'NONE',  ( -62.06710100716626499, -2.637635658083895773, 0.1963493119579517165 ) ) ;
#14096=CARTESIAN_POINT ( 'NONE',  ( -62.05964969381223284, -2.667838369614432548, -0.3597575050025147991 ) ) ;
#14109=ORIENTED_EDGE ( 'NONE', *, *, #395, .T. ) ;
#14130=CARTESIAN_POINT ( 'NONE',  ( -61.34999999999997300, -2.399215024517336925, -0.7870147813924887048 ) ) ;
#14152=AXIS2_PLACEMENT_3D ( 'NONE', #9585, #2600, #19550 ) ;
#14157=DIRECTION ( 'NONE',  ( -2.117927888850090838E-16, 0.02490330187381123786, -0.9996898646859343485 ) ) ;
#14164=DIRECTION ( 'NONE',  ( 0.000000000000000000, 0.9996898646859343485, 0.02490330187381123786 ) ) ;
#14188=DIRECTION ( 'NONE',  ( 0.000000000000000000, -0.9996898646859344595, -0.02490330187381124133 ) ) ;
#14191=DIRECTION ( 'NONE',  ( -1.000000000000000000, -3.053848253006669023E-16, 2.042510438544995169E-16 ) ) ;
#14198=CARTESIAN_POINT ( 'NONE',  ( -60.59999999999998010, -2.482306123512481477, -1.062147028039162944 ) ) ;
#14211=ORIENTED_EDGE ( 'NONE', *, *, #427, .T. ) ;
#14231=CIRCLE ( 'NONE', #13207, 2.625000000000000444 ) ;
#14234=CARTESIAN_POINT ( 'NONE',  ( -62.04999999999998295, -2.687391533643780139, 0.2606275981160435240 ) ) ;
#14238=( BOUNDED_CURVE ( )  B_SPLINE_CURVE ( 3, ( #4665, #21470, #28896, #23841 ),
 .UNSPECIFIED., .F., .T. ) 
 B_SPLINE_CURVE_WITH_KNOTS ( ( 4, 4 ),
 ( 5.004066724468453131, 5.113639620782133299 ),
 .UNSPECIFIED. ) 
 CURVE ( )  GEOMETRIC_REPRESENTATION_ITEM ( )  RATIONAL_B_SPLINE_CURVE ( ( 1.000000000000000000, 0.9989997319336324511, 0.9989997319336324511, 1.000000000000000000 ) ) 
 REPRESENTATION_ITEM ( '' )  );
#14242=CYLINDRICAL_SURFACE ( 'NONE', #5296, 0.4600000000000000755 ) ;
#14244=CIRCLE ( 'NONE', #28400, 2.700000000000000178 ) ;
#14245=CARTESIAN_POINT ( 'NONE',  ( -61.34573509928848978, -2.599898133715064841, 0.4599265640150483336 ) ) ;
#14250=CARTESIAN_POINT ( 'NONE',  ( -74.38999999999998636, -1.239615432210561474, -0.03088009432352123093 ) ) ;
#14263=EDGE_CURVE ( 'NONE', #11253, #4710, #29703, .T. ) ;
#14277=B_SPLINE_CURVE_WITH_KNOTS ( 'NONE', 3,
 ( #19420, #10682, #5625, #30141, #10536, #27459, #15275, #29683, #13200, #17500, #7824, #22884, #27312, #702, #1175, #20366, #24921, #25078, #3240, #20675, #5774, #15426 ),
 .UNSPECIFIED., .F., .F.,
 ( 4, 3, 3, 3, 3, 3, 3, 4 ),
 ( 0.000000000000000000, 1.399909030954194845E-05, 2.803893251624930971E-05, 4.349111487736998725E-05, 6.146574527255033334E-05, 8.260060575193124254E-05, 8.548435886018167966E-05, 8.696130784903155486E-05 ),
 .UNSPECIFIED. ) ;
#14283=CARTESIAN_POINT ( 'NONE',  ( -60.83824777938995965, -2.520112425590160576, -0.9763468200406411057 ) ) ;
#14324=DIRECTION ( 'NONE',  ( -2.117927888850090838E-16, 0.02490330187381123786, -0.9996898646859343485 ) ) ;
#14336=CARTESIAN_POINT ( 'NONE',  ( -62.39999999999998437, 2.699162634652023662, 0.06723891505929276147 ) ) ;
#14345=DIRECTION ( 'NONE',  ( -1.000000000000000000, -3.053848253006669023E-16, 2.042510438544995415E-16 ) ) ;
#14347=LINE ( 'NONE', #23722, #11418 ) ;
#14399=CARTESIAN_POINT ( 'NONE',  ( -62.09999999999998010, -2.671081280896091759, -0.3941126626315458181 ) ) ;
#14426=ORIENTED_EDGE ( 'NONE', *, *, #18783, .F. ) ;
#14445=CARTESIAN_POINT ( 'NONE',  ( -61.34999999999997300, -2.583824419212624957, -0.5885162450438690129 ) ) ;
#14478=EDGE_LOOP ( 'NONE', ( #30265, #6838, #25789, #15676 ) ) ;
#14488=B_SPLINE_CURVE_WITH_KNOTS ( 'NONE', 3,
 ( #22038, #966, #636, #3171 ),
 .UNSPECIFIED., .F., .F.,
 ( 4, 4 ),
 ( 0.000000000000000000, 9.751079247351165789E-06 ),
 .UNSPECIFIED. ) ;
#14491=EDGE_LOOP ( 'NONE', ( #14910, #20278, #29675, #5367 ) ) ;
#14495=EDGE_LOOP ( 'NONE', ( #29956, #21311, #26390, #18725, #23174, #21314 ) ) ;
#14514=EDGE_CURVE ( 'NONE', #1831, #29552, #27146, .T. ) ;
#14526=FACE_OUTER_BOUND ( 'NONE', #13238, .T. ) ;
#14543=DIRECTION ( 'NONE',  ( 0.000000000000000000, -0.9996898646859343485, -0.02490330187381123786 ) ) ;
#14546=CIRCLE ( 'NONE', #8984, 0.01000000000000001929 ) ;
#14566=CARTESIAN_POINT ( 'NONE',  ( -62.05111114591711896, -2.687659336528080534, 0.2567748417330854016 ) ) ;
#14576=CARTESIAN_POINT ( 'NONE',  ( -60.59999999999998010, -2.482306123512481477, -1.062147028039162944 ) ) ;
#14580=ORIENTED_EDGE ( 'NONE', *, *, #14969, .T. ) ;
#14583=VERTEX_POINT ( 'NONE', #18079 ) ;
#14626=ORIENTED_EDGE ( 'NONE', *, *, #15779, .F. ) ;
#14641=AXIS2_PLACEMENT_3D ( 'NONE', #25471, #6316, #25325 ) ;
#14646=CYLINDRICAL_SURFACE ( 'NONE', #19049, 2.700000000000000178 ) ;
#14661=ORIENTED_EDGE ( 'NONE', *, *, #30793, .F. ) ;
#14666=EDGE_CURVE ( 'NONE', #30371, #11715, #25629, .T. ) ;
#14713=DIRECTION ( 'NONE',  ( 0.000000000000000000, -0.9996898646859343485, -0.02490330187381124133 ) ) ;
#14716=EDGE_CURVE ( 'NONE', #30753, #4710, #4907, .T. ) ;
#14740=EDGE_LOOP ( 'NONE', ( #14661, #5024, #7832, #28092 ) ) ;
#14756=EDGE_CURVE ( 'NONE', #6272, #20516, #8433, .T. ) ;
#14771=DIRECTION ( 'NONE',  ( 0.000000000000000000, 0.9996898646859344595, 0.02490330187381119623 ) ) ;
#14786=ADVANCED_FACE ( 'NONE', ( #26126 ), #25652, .T. ) ;
#14804=DIRECTION ( 'NONE',  ( 3.002035892788117459E-16, -0.9996898646859344595, -0.02490330187381123786 ) ) ;
#14818=AXIS2_PLACEMENT_3D ( 'NONE', #20161, #29790, #8105 ) ;
#14834=CARTESIAN_POINT ( 'NONE',  ( -61.84501029485813461, -2.660356430927216298, -0.4698869684439438976 ) ) ;
#14861=ORIENTED_EDGE ( 'NONE', *, *, #19438, .T. ) ;
#14872=DIRECTION ( 'NONE',  ( -3.002035892788116966E-16, 0.9996898646859343485, 0.02490330187381124133 ) ) ;
#14875=ORIENTED_EDGE ( 'NONE', *, *, #7097, .T. ) ;
#14909=CARTESIAN_POINT ( 'NONE',  ( -61.35733863216196227, -2.634673853764536222, 0.4689153067231007777 ) ) ;
#14910=ORIENTED_EDGE ( 'NONE', *, *, #22387, .F. ) ;
#14916=VERTEX_POINT ( 'NONE', #15020 ) ;
#14917=DIRECTION ( 'NONE',  ( -1.000000000000000000, -3.053848253006669023E-16, 2.042510438544995415E-16 ) ) ;
#14924=EDGE_CURVE ( 'NONE', #10954, #13383, #30509, .T. ) ;
#14925=CIRCLE ( 'NONE', #26577, 2.525000000000001688 ) ;
#14969=EDGE_CURVE ( 'NONE', #3863, #21049, #2206, .T. ) ;
#14971=AXIS2_PLACEMENT_3D ( 'NONE', #17361, #5021, #29391 ) ;
#14976=AXIS2_PLACEMENT_3D ( 'NONE', #4668, #11961, #26515 ) ;
#15004=DIRECTION ( 'NONE',  ( -1.000000000000000000, -3.053848253006669023E-16, 2.042510438544995415E-16 ) ) ;
#15008=EDGE_CURVE ( 'NONE', #25398, #66, #27215, .T. ) ;
#15020=CARTESIAN_POINT ( 'NONE',  ( -61.34999999999997300, -2.399215024517336925, -0.7870147813924887048 ) ) ;
#15033=CIRCLE ( 'NONE', #17580, 2.800000000000000266 ) ;
#15041=PLANE ( 'NONE',  #28528 ) ;
#15047=CIRCLE ( 'NONE', #15548, 2.625000000000000444 ) ;
#15053=ADVANCED_FACE ( 'NONE', ( #14526 ), #7883, .T. ) ;
#15065=AXIS2_PLACEMENT_3D ( 'NONE', #28413, #28258, #23500 ) ;
#15078=ORIENTED_EDGE ( 'NONE', *, *, #6783, .T. ) ;
#15084=DIRECTION ( 'NONE',  ( 0.000000000000000000, -0.9996898646859343485, -0.02490330187381116153 ) ) ;
#15100=B_SPLINE_CURVE_WITH_KNOTS ( 'NONE', 3,
 ( #6385, #580, #19909, #14445 ),
 .UNSPECIFIED., .F., .F.,
 ( 4, 4 ),
 ( 0.000000000000000000, 9.751079247352095831E-06 ),
 .UNSPECIFIED. ) ;
#15107=CARTESIAN_POINT ( 'NONE',  ( -61.34999999999997300, -2.528827883897363904, -0.7921676171260561006 ) ) ;
#15113=VECTOR ( 'NONE', #22729, 1000.000000000000000 ) ;
#15122=DIRECTION ( 'NONE',  ( 0.000000000000000000, 0.9996898646859343485, 0.02490330187381123786 ) ) ;
#15125=ORIENTED_EDGE ( 'NONE', *, *, #15478, .F. ) ;
#15141=PRODUCT_DEFINITION ( 'UNKNOWN', '', #3504, #12334 ) ;
#15152=ORIENTED_EDGE ( 'NONE', *, *, #10648, .T. ) ;
#15166=CARTESIAN_POINT ( 'NONE',  ( -60.59999999999998010, -2.408745774756101188, -1.060314564156378037 ) ) ;
#15169=DIRECTION ( 'NONE',  ( 3.002035892788117459E-16, -0.9996898646859343485, -0.02490330187381124480 ) ) ;
#15173=CARTESIAN_POINT ( 'NONE',  ( -61.39999999999998437, -2.624491116890564690, -0.6340712715164679159 ) ) ;
#15217=DIRECTION ( 'NONE',  ( -2.117927888850090838E-16, 0.02490330187381123786, -0.9996898646859343485 ) ) ;
#15225=LINE ( 'NONE', #17153, #27609 ) ;
#15236=CARTESIAN_POINT ( 'NONE',  ( -60.63087243001902493, -2.460428303538280570, -1.102619274812461025 ) ) ;
#15254=DIRECTION ( 'NONE',  ( -1.000000000000000000, -3.053848253006669023E-16, 2.042510438544995415E-16 ) ) ;
#15263=DIRECTION ( 'NONE',  ( -3.002035892788117459E-16, 0.9996898646859344595, 0.02490330187381124133 ) ) ;
#15274=FACE_OUTER_BOUND ( 'NONE', #30967, .T. ) ;
#15275=CARTESIAN_POINT ( 'NONE',  ( -61.35738992240673184, -2.589110738181390037, 0.6770092922617376718 ) ) ;
#15297=CARTESIAN_POINT ( 'NONE',  ( -62.07183734345855441, -2.637794457623054534, 0.1946209358647623400 ) ) ;
#15322=DIRECTION ( 'NONE',  ( 0.000000000000000000, 0.9996898646859343485, 0.02490330187381123786 ) ) ;
#15328=ADVANCED_FACE ( 'NONE', ( #3890 ), #20069, .F. ) ;
#15346=CARTESIAN_POINT ( 'NONE',  ( -61.34999999999997300, -2.617575446388284099, 0.6620413751912884726 ) ) ;
#15348=ORIENTED_EDGE ( 'NONE', *, *, #7930, .T. ) ;
#15368=AXIS2_PLACEMENT_3D ( 'NONE', #22294, #1315, #30292 ) ;
#15385=FACE_OUTER_BOUND ( 'NONE', #16292, .T. ) ;
#15402=ADVANCED_FACE ( 'NONE', ( #7529 ), #19728, .T. ) ;
#15426=CARTESIAN_POINT ( 'NONE',  ( -61.39999999999998437, -2.604492677689918878, 0.7117709546332967596 ) ) ;
#15436=EDGE_CURVE ( 'NONE', #16145, #2467, #20572, .T. ) ;
#15439=CARTESIAN_POINT ( 'NONE',  ( -61.34999999999997300, -2.551764585593653489, 0.6636807913650824009 ) ) ;
#15473=DIRECTION ( 'NONE',  ( 1.000000000000000000, 3.053848253006669023E-16, -2.042510438544995415E-16 ) ) ;
#15478=EDGE_CURVE ( 'NONE', #29552, #18413, #28211, .T. ) ;
#15483=CIRCLE ( 'NONE', #18023, 2.625000000000000444 ) ;
#15487=CARTESIAN_POINT ( 'NONE',  ( -61.82615520548803545, -2.612112197326142304, -0.4148502322964471856 ) ) ;
#15491=TOROIDAL_SURFACE ( 'NONE', #5863, 1.239999999999999991, 0.01000000000000000021 ) ;
#15503=ORIENTED_EDGE ( 'NONE', *, *, #2074, .F. ) ;
#15517=DIRECTION ( 'NONE',  ( 1.000000000000000000, 3.053848253006669023E-16, -2.042510438544995415E-16 ) ) ;
#15534=CYLINDRICAL_SURFACE ( 'NONE', #12413, 1.250000000000000222 ) ;
#15536=CIRCLE ( 'NONE', #1885, 0.04999999999999988481 ) ;
#15541=CARTESIAN_POINT ( 'NONE',  ( -62.08600056051449201, -2.518032341469984559, 0.1874854198766372493 ) ) ;
#15544=CARTESIAN_POINT ( 'NONE',  ( -62.09999999999997300, -2.706459356064251587, -0.3286898414610474606 ) ) ;
#15548=AXIS2_PLACEMENT_3D ( 'NONE', #4216, #9146, #16413 ) ;
#15585=CARTESIAN_POINT ( 'NONE',  ( -60.59999999999997300, -2.342723651847746336, 0.9419505778294103848 ) ) ;
#15612=CARTESIAN_POINT ( 'NONE',  ( -73.84999999999996589, 1.301636140808604125, 0.03242509391110787870 ) ) ;
#15615=CARTESIAN_POINT ( 'NONE',  ( -44.49999999999997868, 6.542789527549899840E-15, -1.397091617737396343E-15 ) ) ;
#15625=( GEOMETRIC_REPRESENTATION_CONTEXT ( 3 ) GLOBAL_UNCERTAINTY_ASSIGNED_CONTEXT ( ( #17408 ) ) GLOBAL_UNIT_ASSIGNED_CONTEXT ( ( #5905, #25041, #7792 ) ) REPRESENTATION_CONTEXT ( 'NONE', 'WORKASPACE' ) );
#15630=ORIENTED_EDGE ( 'NONE', *, *, #21367, .F. ) ;
#15634=ORIENTED_EDGE ( 'NONE', *, *, #6103, .T. ) ;
#15640=ADVANCED_FACE ( 'NONE', ( #11273 ), #8447, .T. ) ;
#15662=ADVANCED_FACE ( 'NONE', ( #25384 ), #16204, .T. ) ;
#15676=ORIENTED_EDGE ( 'NONE', *, *, #24341, .F. ) ;
#15677=DIRECTION ( 'NONE',  ( 0.3420201433256666590, 0.02340144900402443481, -0.9394011889198365939 ) ) ;
#15681=DIRECTION ( 'NONE',  ( 1.000000000000000000, 3.053848253006669023E-16, -2.042510438544995415E-16 ) ) ;
#15701=CARTESIAN_POINT ( 'NONE',  ( -62.34999999999997300, 2.799131621120618085, 0.06972924524667374613 ) ) ;
#15711=CARTESIAN_POINT ( 'NONE',  ( -60.64918514029853469, -2.458741238023958608, -1.115600605136573220 ) ) ;
#15722=ORIENTED_EDGE ( 'NONE', *, *, #2208, .T. ) ;
#15728=CARTESIAN_POINT ( 'NONE',  ( -61.82620411128901594, -2.510158248709655648, 0.2872314057388253294 ) ) ;
#15734=DIRECTION ( 'NONE',  ( 0.3420201433256677137, -0.02340144900402421971, 0.9394011889198362608 ) ) ;
#15735=DIRECTION ( 'NONE',  ( 1.000000000000000000, 3.053848253006669023E-16, -2.042510438544995415E-16 ) ) ;
#15740=CARTESIAN_POINT ( 'NONE',  ( -62.06710100716625789, -2.637635658083895329, 0.1963493119579511614 ) ) ;
#15773=AXIS2_PLACEMENT_3D ( 'NONE', #11480, #21163, #30794 ) ;
#15779=EDGE_CURVE ( 'NONE', #23465, #6272, #10962, .T. ) ;
#15791=DIRECTION ( 'NONE',  ( 0.000000000000000000, 0.9996898646859344595, 0.02490330187381124133 ) ) ;
#15805=EDGE_CURVE ( 'NONE', #5852, #23537, #9474, .T. ) ;
#15813=ORIENTED_EDGE ( 'NONE', *, *, #30919, .T. ) ;
#15834=EDGE_CURVE ( 'NONE', #4977, #13516, #8762, .T. ) ;
#15866=CIRCLE ( 'NONE', #17384, 2.750000000000000444 ) ;
#15879=AXIS2_PLACEMENT_3D ( 'NONE', #626, #12971, #10287 ) ;
#15883=ORIENTED_EDGE ( 'NONE', *, *, #19502, .T. ) ;
#15890=ORIENTED_EDGE ( 'NONE', *, *, #24864, .T. ) ;
#15896=DIRECTION ( 'NONE',  ( -1.000000000000000000, -3.053848253006669023E-16, 2.042510438544995415E-16 ) ) ;
#15898=B_SPLINE_CURVE_WITH_KNOTS ( 'NONE', 3,
 ( #30114, #27130, #13180, #8278 ),
 .UNSPECIFIED., .F., .F.,
 ( 4, 4 ),
 ( 0.000000000000000000, 1.346394374510315309E-05 ),
 .UNSPECIFIED. ) ;
#15901=DIRECTION ( 'NONE',  ( 0.000000000000000000, -0.9996898646859343485, -0.02490330187381124133 ) ) ;
#15944=TOROIDAL_SURFACE ( 'NONE', #21539, 1.302039949377232331, 0.05000000000000000278 ) ;
#15948=CIRCLE ( 'NONE', #27568, 0.4600000000000000755 ) ;
#15956=EDGE_LOOP ( 'NONE', ( #24323, #27223, #25435, #30814 ) ) ;
#15963=AXIS2_PLACEMENT_3D ( 'NONE', #8994, #11536, #18664 ) ;
#15989=DIRECTION ( 'NONE',  ( 1.000000000000000000, 3.053848253006669023E-16, -2.042510438544995415E-16 ) ) ;
#16000=AXIS2_PLACEMENT_3D ( 'NONE', #18854, #4432, #6494 ) ;
#16001=CARTESIAN_POINT ( 'NONE',  ( -62.05596007256994540, -2.671012538737645770, -0.3731730811386074209 ) ) ;
#16037=DIRECTION ( 'NONE',  ( 1.000000000000000000, 3.053848253006669023E-16, -2.042510438544995415E-16 ) ) ;
#16042=AXIS2_PLACEMENT_3D ( 'NONE', #9659, #12023, #21530 ) ;
#16057=ORIENTED_EDGE ( 'NONE', *, *, #13490, .F. ) ;
#16122=AXIS2_PLACEMENT_3D ( 'NONE', #2906, #22083, #17316 ) ;
#16130=CARTESIAN_POINT ( 'NONE',  ( -64.28602961791190751, 2.263268244922573835, 0.05638033785850931484 ) ) ;
#16145=VERTEX_POINT ( 'NONE', #6257 ) ;
#16165=CIRCLE ( 'NONE', #14152, 2.750000000000000444 ) ;
#16183=EDGE_LOOP ( 'NONE', ( #5498, #30376, #25427, #13015 ) ) ;
#16189=EDGE_LOOP ( 'NONE', ( #7053, #2980, #26453, #6474 ) ) ;
#16193=CIRCLE ( 'NONE', #2037, 2.525000000000001243 ) ;
#16198=DIRECTION ( 'NONE',  ( 0.000000000000000000, 0.9996898646859344595, 0.02490330187381124133 ) ) ;
#16202=EDGE_CURVE ( 'NONE', #3831, #23278, #4627, .T. ) ;
#16204=PLANE ( 'NONE',  #12946 ) ;
#16217=CARTESIAN_POINT ( 'NONE',  ( -63.82928932188132620, 6.399178848011186396E-16, 2.550935903222500290E-15 ) ) ;
#16250=ORIENTED_EDGE ( 'NONE', *, *, #20575, .T. ) ;
#16270=EDGE_CURVE ( 'NONE', #25398, #7079, #15948, .T. ) ;
#16292=EDGE_LOOP ( 'NONE', ( #7659, #5004, #28262, #8614, #9687 ) ) ;
#16300=DIRECTION ( 'NONE',  ( 0.000000000000000000, -0.9996898646859344595, -0.02490330187381124480 ) ) ;
#16317=EDGE_CURVE ( 'NONE', #28072, #2901, #13397, .T. ) ;
#16338=ORIENTED_EDGE ( 'NONE', *, *, #11524, .T. ) ;
#16350=CARTESIAN_POINT ( 'NONE',  ( -61.40479058095097287, -2.566399095993047830, -0.8388061039871230751 ) ) ;
#16377=ORIENTED_EDGE ( 'NONE', *, *, #15436, .T. ) ;
#16379=CYLINDRICAL_SURFACE ( 'NONE', #27836, 2.525000000000001243 ) ;
#16381=DIRECTION ( 'NONE',  ( 0.000000000000000000, 0.9996898646859344595, 0.02490330187381124133 ) ) ;
#16385=CARTESIAN_POINT ( 'NONE',  ( -62.09999999999997300, -2.718470093012312905, 0.1920549639088918459 ) ) ;
#16410=DIRECTION ( 'NONE',  ( 0.000000000000000000, 0.9996898646859343485, 0.02490330187381116153 ) ) ;
#16413=DIRECTION ( 'NONE',  ( 0.000000000000000000, -0.9996898646859344595, -0.02490330187381124480 ) ) ;
#16432=EDGE_CURVE ( 'NONE', #2467, #16145, #24058, .T. ) ;
#16449=DIRECTION ( 'NONE',  ( -1.000000000000000000, -3.053848253006669023E-16, 2.042510438544995415E-16 ) ) ;
#16477=CARTESIAN_POINT ( 'NONE',  ( -62.05403641351750821, -2.672098272234639804, -0.3800858690569366982 ) ) ;
#16479=DIRECTION ( 'NONE',  ( 1.000000000000000000, 3.053848253006669023E-16, -2.042510438544995415E-16 ) ) ;
#16480=CARTESIAN_POINT ( 'NONE',  ( -73.89999999999997726, 1.259609229504275341, 0.03137816036100692790 ) ) ;
#16512=VECTOR ( 'NONE', #5882, 999.9999999999998863 ) ;
#16520=ORIENTED_EDGE ( 'NONE', *, *, #15834, .T. ) ;
#16546=CARTESIAN_POINT ( 'NONE',  ( -62.14999999999998437, -2.749147127886318653, -0.06848408015297871576 ) ) ;
#16548=AXIS2_PLACEMENT_3D ( 'NONE', #685, #22251, #10344 ) ;
#16549=CARTESIAN_POINT ( 'NONE',  ( -60.59999999999997300, 1.626093840209163176E-15, 1.891350188320046374E-15 ) ) ;
#16557=AXIS2_PLACEMENT_3D ( 'NONE', #29302, #12808, #24538 ) ;
#16572=VECTOR ( 'NONE', #5195, 1000.000000000000000 ) ;
#16575=ORIENTED_EDGE ( 'NONE', *, *, #25114, .F. ) ;
#16584=EDGE_LOOP ( 'NONE', ( #20515, #3054, #30617, #22138 ) ) ;
#16587=EDGE_LOOP ( 'NONE', ( #27576, #14109 ) ) ;
#16589=EDGE_CURVE ( 'NONE', #24092, #21049, #14238, .T. ) ;
#16597=CIRCLE ( 'NONE', #18110, 2.700000000000000178 ) ;
#16622=ORIENTED_EDGE ( 'NONE', *, *, #16787, .F. ) ;
#16635=CARTESIAN_POINT ( 'NONE',  ( -61.37588895521345478, -2.622661570964761157, -0.6163042711484312264 ) ) ;
#16646=FACE_OUTER_BOUND ( 'NONE', #28116, .T. ) ;
#16651=CARTESIAN_POINT ( 'NONE',  ( -62.04999999999998295, -2.671081280896084653, -0.3941126626315447634 ) ) ;
#16682=LINE ( 'NONE', #1610, #10915 ) ;
#16715=EDGE_CURVE ( 'NONE', #20326, #26621, #13932, .T. ) ;
#16726=PRODUCT ( 'Twister Head', 'Twister Head', '', ( #18688 ) ) ;
#16747=DIRECTION ( 'NONE',  ( 3.002035892788117459E-16, -0.9996898646859343485, -0.02490330187381123786 ) ) ;
#16760=ORIENTED_EDGE ( 'NONE', *, *, #27808, .T. ) ;
#16782=DIRECTION ( 'NONE',  ( 1.738188194345512309E-16, 0.09652874004297619381, 0.9953301976458442946 ) ) ;
#16783=CIRCLE ( 'NONE', #9205, 1.240000000000000213 ) ;
#16785=CARTESIAN_POINT ( 'NONE',  ( -61.35212117932173470, -2.597517021324610820, -0.5932794490111470420 ) ) ;
#16787=EDGE_CURVE ( 'NONE', #27015, #26621, #7806, .T. ) ;
#16790=ORIENTED_EDGE ( 'NONE', *, *, #10347, .T. ) ;
#16813=ORIENTED_EDGE ( 'NONE', *, *, #20982, .F. ) ;
#16817=ADVANCED_FACE ( 'NONE', ( #2612 ), #15491, .T. ) ;
#16890=DIRECTION ( 'NONE',  ( 0.000000000000000000, -0.9996898646859343485, -0.02490330187381124133 ) ) ;
#16905=CIRCLE ( 'NONE', #3244, 2.800000000000000266 ) ;
#16915=CARTESIAN_POINT ( 'NONE',  ( -67.33025350686975230, -2.149980434289362918, -0.05355822207391593842 ) ) ;
#16946=EDGE_CURVE ( 'NONE', #2594, #30944, #30641, .T. ) ;
#16947=CARTESIAN_POINT ( 'NONE',  ( -62.05677242593181120, -2.685607875047633541, 0.2368181935235877944 ) ) ;
#16948=CIRCLE ( 'NONE', #5821, 0.04999999999999988481 ) ;
#16984=EDGE_CURVE ( 'NONE', #24287, #20326, #16682, .T. ) ;
#17012=CIRCLE ( 'NONE', #18543, 1.250000000000000222 ) ;
#17018=ORIENTED_EDGE ( 'NONE', *, *, #14716, .F. ) ;
#17019=CIRCLE ( 'NONE', #7393, 0.04999999999999988481 ) ;
#17020=FACE_OUTER_BOUND ( 'NONE', #14491, .T. ) ;
#17021=DIRECTION ( 'NONE',  ( 3.002035892788117459E-16, -0.9996898646859343485, -0.02490330187381123786 ) ) ;
#17030=CARTESIAN_POINT ( 'NONE',  ( -44.49999999999997868, 6.542789527549899840E-15, -1.397091617737396343E-15 ) ) ;
#17044=B_SPLINE_CURVE_WITH_KNOTS ( 'NONE', 3,
 ( #24268, #21908, #12226, #2721, #22212, #500, #22358, #190, #7632, #17438, #7483, #24557, #12363, #3033, #2878, #29457, #24720, #648, #26475 ),
 .UNSPECIFIED., .F., .F.,
 ( 4, 3, 3, 3, 3, 3, 4 ),
 ( -1.476948988848390564E-06, 2.117582368135750848E-22, 2.236146517042047793E-05, 4.055096472349869428E-05, 5.611001533034534733E-05, 7.070124744307527942E-05, 8.536389545014277545E-05 ),
 .UNSPECIFIED. ) ;
#17070=EDGE_CURVE ( 'NONE', #28721, #3863, #12425, .T. ) ;
#17082=LINE ( 'NONE', #2506, #15113 ) ;
#17088=ORIENTED_EDGE ( 'NONE', *, *, #21367, .T. ) ;
#17146=CARTESIAN_POINT ( 'NONE',  ( -67.36397038208805554, -4.395200732636863594E-16, 3.272898199462452353E-15 ) ) ;
#17153=CARTESIAN_POINT ( 'NONE',  ( -73.89999999999997726, 1.349581317326009389, 0.03361945752964979467 ) ) ;
#17178=ORIENTED_EDGE ( 'NONE', *, *, #12134, .T. ) ;
#17184=CARTESIAN_POINT ( 'NONE',  ( -60.49999999999997868, -2.624185894800576957, -0.06537116741875233228 ) ) ;
#17210=ORIENTED_EDGE ( 'NONE', *, *, #15436, .F. ) ;
#17233=CARTESIAN_POINT ( 'NONE',  ( -61.58548216437489486, -2.595212895210543991, -0.5020542520759796457 ) ) ;
#17269=ADVANCED_FACE ( 'NONE', ( #10768 ), #15534, .T. ) ;
#17272=DIRECTION ( 'NONE',  ( -1.000000000000000000, -3.053848253006669023E-16, 2.042510438544995415E-16 ) ) ;
#17295=CARTESIAN_POINT ( 'NONE',  ( -62.09999999999997300, -2.634806471255679572, -0.2806920565413739133 ) ) ;
#17298=LINE ( 'NONE', #29015, #11910 ) ;
#17316=DIRECTION ( 'NONE',  ( 0.000000000000000000, -0.9996898646859344595, -0.02490330187381124480 ) ) ;
#17331=DIRECTION ( 'NONE',  ( 0.000000000000000000, 0.9996898646859344595, 0.02490330187381124133 ) ) ;
#17344=EDGE_LOOP ( 'NONE', ( #9104, #14211, #8995, #22576 ) ) ;
#17361=CARTESIAN_POINT ( 'NONE',  ( -62.39999999999998437, 1.076401154667962023E-15, 2.259002067258145746E-15 ) ) ;
#17384=AXIS2_PLACEMENT_3D ( 'NONE', #20167, #3361, #25358 ) ;
#17408=UNCERTAINTY_MEASURE_WITH_UNIT (LENGTH_MEASURE( 1.000000000000000082E-05 ), #5905, 'distance_accuracy_value', 'NONE');
#17430=CARTESIAN_POINT ( 'NONE',  ( -62.39999999999998437, 1.076401154667962023E-15, 2.259002067258145746E-15 ) ) ;
#17436=DIRECTION ( 'NONE',  ( -1.000000000000000000, -3.053848253006669023E-16, 2.042510438544995415E-16 ) ) ;
#17438=CARTESIAN_POINT ( 'NONE',  ( -61.36734273774667514, -2.561240237610082904, -0.8152598366033302346 ) ) ;
#17459=ORIENTED_EDGE ( 'NONE', *, *, #19545, .F. ) ;
#17491=ORIENTED_EDGE ( 'NONE', *, *, #10095, .T. ) ;
#17492=CIRCLE ( 'NONE', #15963, 1.240000000000000213 ) ;
#17497=CARTESIAN_POINT ( 'NONE',  ( -62.08111617280007266, -2.505022497657029223, -0.3170112821859903951 ) ) ;
#17499=DIRECTION ( 'NONE',  ( -1.000000000000000000, -3.053848253006669023E-16, 2.042510438544995169E-16 ) ) ;
#17500=CARTESIAN_POINT ( 'NONE',  ( -61.36641165373034568, -2.598025853916357431, 0.6858830576151544456 ) ) ;
#17524=ADVANCED_FACE ( 'NONE', ( #16646 ), #14242, .F. ) ;
#17530=STYLED_ITEM ( 'NONE', ( #26326 ), #26054 ) ;
#17543=CARTESIAN_POINT ( 'NONE',  ( -61.82074345547174232, -2.669507762876991208, -0.4182503418061432332 ) ) ;
#17553=DIRECTION ( 'NONE',  ( -1.000000000000000000, -3.053848253006669023E-16, 2.042510438544995415E-16 ) ) ;
#17563=ORIENTED_EDGE ( 'NONE', *, *, #1150, .F. ) ;
#17580=AXIS2_PLACEMENT_3D ( 'NONE', #29890, #29561, #24823 ) ;
#17588=ORIENTED_EDGE ( 'NONE', *, *, #17953, .T. ) ;
#17606=CARTESIAN_POINT ( 'NONE',  ( -61.34999999999997300, 1.397055221233662433E-15, 2.044538471210920981E-15 ) ) ;
#17627=ORIENTED_EDGE ( 'NONE', *, *, #20575, .F. ) ;
#17665=CARTESIAN_POINT ( 'NONE',  ( -61.34999999999997300, -2.551764585593653489, 0.6636807913650824009 ) ) ;
#17683=( GEOMETRIC_REPRESENTATION_CONTEXT ( 3 ) GLOBAL_UNCERTAINTY_ASSIGNED_CONTEXT ( ( #7904 ) ) GLOBAL_UNIT_ASSIGNED_CONTEXT ( ( #13777, #18405, #11258 ) ) REPRESENTATION_CONTEXT ( 'NONE', 'WORKASPACE' ) );
#17687=CARTESIAN_POINT ( 'NONE',  ( -62.09999999999997300, 1.168016602258162478E-15, 2.197726754101795588E-15 ) ) ;
#17689=AXIS2_PLACEMENT_3D ( 'NONE', #29961, #14917, #27278 ) ;
#17705=CARTESIAN_POINT ( 'NONE',  ( -60.64999999999998437, -2.458515422985869670, -1.116110171506649040 ) ) ;
#17710=CIRCLE ( 'NONE', #8581, 2.700000000000000178 ) ;
#17719=AXIS2_PLACEMENT_3D ( 'NONE', #15612, #1638, #17832 ) ;
#17720=CARTESIAN_POINT ( 'NONE',  ( -74.39999999999997726, 1.249612330857415632, 0.03112912734226876837 ) ) ;
#17722=DIRECTION ( 'NONE',  ( -3.002035892788117459E-16, 0.9996898646859344595, 0.02490330187381124133 ) ) ;
#17725=AXIS2_PLACEMENT_3D ( 'NONE', #30947, #27938, #25725 ) ;
#17727=CARTESIAN_POINT ( 'NONE',  ( -60.64959257988790853, -2.511140837076556220, 0.9920543200944375029 ) ) ;
#17780=CARTESIAN_POINT ( 'NONE',  ( -60.62613029541262222, -2.459964683042519695, -1.098852628973487233 ) ) ;
#17800=CIRCLE ( 'NONE', #3109, 2.525000000000001243 ) ;
#17802=DIRECTION ( 'NONE',  ( 0.000000000000000000, -0.9996898646859343485, -0.02490330187381124133 ) ) ;
#17832=DIRECTION ( 'NONE',  ( 0.000000000000000000, -0.9996898646859344595, -0.02490330187381133153 ) ) ;
#17862=ORIENTED_EDGE ( 'NONE', *, *, #27443, .F. ) ;
#17872=VECTOR ( 'NONE', #21258, 999.9999999999998863 ) ;
#17884=CYLINDRICAL_SURFACE ( 'NONE', #11805, 0.4600000000000000755 ) ;
#17920=CARTESIAN_POINT ( 'NONE',  ( -73.85208152723558328, -1.351577301140755472, -0.03366917953766473959 ) ) ;
#17953=EDGE_CURVE ( 'NONE', #28678, #8829, #6381, .T. ) ;
#17955=EDGE_CURVE ( 'NONE', #18759, #1827, #7321, .T. ) ;
#17965=CARTESIAN_POINT ( 'NONE',  ( -67.89999999999997726, -6.032153844857049047E-16, 3.382382808457892732E-15 ) ) ;
#18013=DIRECTION ( 'NONE',  ( 0.000000000000000000, 0.9996898646859343485, 0.02490330187381124133 ) ) ;
#18021=CARTESIAN_POINT ( 'NONE',  ( -61.34999999999997300, 1.397055221233662433E-15, 2.044538471210920981E-15 ) ) ;
#18023=AXIS2_PLACEMENT_3D ( 'NONE', #9643, #26405, #9777 ) ;
#18026=LINE ( 'NONE', #13245, #20020 ) ;
#18058=CARTESIAN_POINT ( 'NONE',  ( -62.09999999999997300, -2.720545749060828022, -0.4014110452728629763 ) ) ;
#18073=AXIS2_PLACEMENT_3D ( 'NONE', #6243, #28689, #25544 ) ;
#18079=CARTESIAN_POINT ( 'NONE',  ( -60.49999999999997868, -2.524216908331982978, -0.06288083723137102843 ) ) ;
#18085=CIRCLE ( 'NONE', #22134, 2.249352573995730520 ) ;
#18088=CARTESIAN_POINT ( 'NONE',  ( -62.09999999999997300, -2.682569912478698804, -0.3012640610164738497 ) ) ;
#18107=ORIENTED_EDGE ( 'NONE', *, *, #26532, .F. ) ;
#18110=AXIS2_PLACEMENT_3D ( 'NONE', #1529, #27968, #14188 ) ;
#18120=CARTESIAN_POINT ( 'NONE',  ( -60.64999999999998437, 1.610824598944129570E-15, 1.901562740512771401E-15 ) ) ;
#18121=CIRCLE ( 'NONE', #2421, 2.700000000000000178 ) ;
#18129=CARTESIAN_POINT ( 'NONE',  ( -62.09999999999997300, 1.168016602258162478E-15, 2.197726754101795588E-15 ) ) ;
#18193=EDGE_CURVE ( 'NONE', #22436, #19955, #17044, .T. ) ;
#18203=AXIS2_PLACEMENT_3D ( 'NONE', #11220, #11701, #9010 ) ;
#18211=CIRCLE ( 'NONE', #6554, 0.04999999999999988481 ) ;
#18236=AXIS2_PLACEMENT_3D ( 'NONE', #4848, #14345, #16747 ) ;
#18247=CARTESIAN_POINT ( 'NONE',  ( -67.89999999999997726, -1.599503783497495890, -0.03984528299809441537 ) ) ;
#18250=ORIENTED_EDGE ( 'NONE', *, *, #13638, .F. ) ;
#18254=CARTESIAN_POINT ( 'NONE',  ( -61.34999999999997300, -2.609922480197373940, 0.4591346723570145505 ) ) ;
#18255=ORIENTED_EDGE ( 'NONE', *, *, #395, .F. ) ;
#18259=AXIS2_PLACEMENT_3D ( 'NONE', #21710, #28958, #19176 ) ;
#18289=ORIENTED_EDGE ( 'NONE', *, *, #9177, .F. ) ;
#18290=ORIENTED_EDGE ( 'NONE', *, *, #10083, .T. ) ;
#18292=ORIENTED_EDGE ( 'NONE', *, *, #23253, .F. ) ;
#18343=CYLINDRICAL_SURFACE ( 'NONE', #19465, 0.05000000000000001665 ) ;
#18356=EDGE_LOOP ( 'NONE', ( #20334, #3375, #6833, #23447 ) ) ;
#18358=DIRECTION ( 'NONE',  ( 3.002035892788116966E-16, -0.9996898646859343485, -0.02490330187381124133 ) ) ;
#18400=LINE ( 'NONE', #28037, #19969 ) ;
#18405=( NAMED_UNIT ( * ) PLANE_ANGLE_UNIT ( ) SI_UNIT ( $, .RADIAN. ) );
#18413=VERTEX_POINT ( 'NONE', #26291 ) ;
#18414=EDGE_CURVE ( 'NONE', #20935, #18759, #23296, .T. ) ;
#18442=VERTEX_POINT ( 'NONE', #13604 ) ;
#18456=DIRECTION ( 'NONE',  ( -1.000000000000000000, -3.053848253006669023E-16, 2.042510438544995415E-16 ) ) ;
#18466=CARTESIAN_POINT ( 'NONE',  ( -61.38137739671037707, -2.621185111045226446, 0.6505274733237536022 ) ) ;
#18468=DIRECTION ( 'NONE',  ( 3.002035892788117459E-16, -0.9996898646859344595, -0.02490330187381123786 ) ) ;
#18485=DIRECTION ( 'NONE',  ( 2.117927888850090591E-16, -0.02490330187381111643, 0.9996898646859343485 ) ) ;
#18498=VECTOR ( 'NONE', #28021, 1000.000000000000114 ) ;
#18522=CARTESIAN_POINT ( 'NONE',  ( -44.49999999999997868, 6.542789527549899840E-15, -1.397091617737396343E-15 ) ) ;
#18543=AXIS2_PLACEMENT_3D ( 'NONE', #25423, #12087, #8636 ) ;
#18550=DIRECTION ( 'NONE',  ( 1.000000000000000000, 3.053848253006669023E-16, -2.042510438544995415E-16 ) ) ;
#18565=CIRCLE ( 'NONE', #21662, 2.750000000000000444 ) ;
#18600=EDGE_LOOP ( 'NONE', ( #2564, #16338, #8712, #1373 ) ) ;
#18602=EDGE_CURVE ( 'NONE', #1827, #1635, #30216, .T. ) ;
#18620=ADVANCED_FACE ( 'NONE', ( #942 ), #1088, .F. ) ;
#18634=ORIENTED_EDGE ( 'NONE', *, *, #16589, .T. ) ;
#18652=ORIENTED_EDGE ( 'NONE', *, *, #7190, .F. ) ;
#18657=DIRECTION ( 'NONE',  ( 0.000000000000000000, 0.9996898646859347926, 0.02490330187379614924 ) ) ;
#18664=DIRECTION ( 'NONE',  ( 0.000000000000000000, -0.9996898646859343485, -0.02490330187381124133 ) ) ;
#18675=FACE_OUTER_BOUND ( 'NONE', #25160, .T. ) ;
#18684=DIRECTION ( 'NONE',  ( 1.000000000000000000, 3.053848253006669023E-16, -2.042510438544995415E-16 ) ) ;
#18688=PRODUCT_CONTEXT ( 'NONE', #4261, 'mechanical' ) ;
#18708=CARTESIAN_POINT ( 'NONE',  ( -62.09999999999997300, -2.665234058423473495, -0.3155123021236101999 ) ) ;
#18710=FACE_OUTER_BOUND ( 'NONE', #23200, .T. ) ;
#18716=LINE ( 'NONE', #18247, #22170 ) ;
#18725=ORIENTED_EDGE ( 'NONE', *, *, #1402, .T. ) ;
#18745=FILL_AREA_STYLE ('',( #30585 ) ) ;
#18759=VERTEX_POINT ( 'NONE', #30681 ) ;
#18776=ORIENTED_EDGE ( 'NONE', *, *, #775, .F. ) ;
#18783=EDGE_CURVE ( 'NONE', #20516, #8800, #17492, .T. ) ;
#18840=CARTESIAN_POINT ( 'NONE',  ( -62.34999999999997300, -2.799131621120615421, -0.06972924524666888890 ) ) ;
#18854=CARTESIAN_POINT ( 'NONE',  ( -67.34999999999998010, -4.352537305703398686E-16, 3.270044734337918230E-15 ) ) ;
#18862=DIRECTION ( 'NONE',  ( 0.000000000000000000, 0.02490330187380866006, -0.9996898646859344595 ) ) ;
#18877=DIRECTION ( 'NONE',  ( 1.000000000000000000, 3.053848253006669023E-16, -2.042510438544995415E-16 ) ) ;
#18895=SURFACE_STYLE_USAGE ( .BOTH. , #13956 ) ;
#18919=ORIENTED_EDGE ( 'NONE', *, *, #22937, .T. ) ;
#18924=DIRECTION ( 'NONE',  ( 1.000000000000000000, 3.053848253006669023E-16, -2.042510438544995415E-16 ) ) ;
#18932=CARTESIAN_POINT ( 'NONE',  ( -62.09999999999997300, -2.647063127320109288, 0.1491152568578474336 ) ) ;
#18969=AXIS2_PLACEMENT_3D ( 'NONE', #25035, #29473, #12695 ) ;
#18990=ORIENTED_EDGE ( 'NONE', *, *, #10588, .T. ) ;
#18998=ADVANCED_FACE ( 'NONE', ( #5171 ), #21585, .F. ) ;
#19006=PLANE ( 'NONE',  #18259 ) ;
#19007=CARTESIAN_POINT ( 'NONE',  ( -62.06826830520247285, -2.668664083165746881, 0.1951513684571901941 ) ) ;
#19010=EDGE_CURVE ( 'NONE', #24287, #27015, #15483, .T. ) ;
#19027=AXIS2_PLACEMENT_3D ( 'NONE', #26862, #4860, #122 ) ;
#19049=AXIS2_PLACEMENT_3D ( 'NONE', #12263, #21948, #19575 ) ;
#19053=CARTESIAN_POINT ( 'NONE',  ( -61.38137739671039128, -2.585543411474696462, -0.7802324315830138080 ) ) ;
#19057=( NAMED_UNIT ( * ) PLANE_ANGLE_UNIT ( ) SI_UNIT ( $, .RADIAN. ) );
#19088=DIRECTION ( 'NONE',  ( 0.000000000000000000, 0.9996898646859344595, 0.02490330187381124133 ) ) ;
#19131=DIRECTION ( 'NONE',  ( 3.002035892788116966E-16, -0.9996898646859343485, -0.02490330187381123786 ) ) ;
#19174=CARTESIAN_POINT ( 'NONE',  ( -61.35552595367609996, -2.605636331997853716, -0.5976426842213763413 ) ) ;
#19176=DIRECTION ( 'NONE',  ( 3.002035892788116966E-16, -0.9996898646859343485, -0.02490330187381123786 ) ) ;
#19255=CARTESIAN_POINT ( 'NONE',  ( -73.89999999999997726, -2.435524336289708093E-15, 4.607889071584891164E-15 ) ) ;
#19294=EDGE_CURVE ( 'NONE', #29446, #3316, #17012, .T. ) ;
#19333=CARTESIAN_POINT ( 'NONE',  ( -62.06004451743454808, -2.681695334896316840, 0.2250289189416591340 ) ) ;
#19348=EDGE_LOOP ( 'NONE', ( #4110, #221, #22116, #20820 ) ) ;
#19353=CARTESIAN_POINT ( 'NONE',  ( -67.91948434493399134, -6.091656077594763675E-16, 3.386362506249485869E-15 ) ) ;
#19363=ORIENTED_EDGE ( 'NONE', *, *, #10083, .F. ) ;
#19377=DIRECTION ( 'NONE',  ( 0.3420201433256648826, 0.02340144900402444869, -0.9394011889198372600 ) ) ;
#19397=FACE_OUTER_BOUND ( 'NONE', #2179, .T. ) ;
#19411=CIRCLE ( 'NONE', #12288, 0.05000000000000009298 ) ;
#19420=CARTESIAN_POINT ( 'NONE',  ( -61.34999999999997300, -2.565134197206211386, 0.6652717868084008224 ) ) ;
#19425=EDGE_CURVE ( 'NONE', #5085, #2901, #15225, .T. ) ;
#19434=AXIS2_PLACEMENT_3D ( 'NONE', #31213, #12207, #14872 ) ;
#19438=EDGE_CURVE ( 'NONE', #28678, #21812, #9023, .T. ) ;
#19465=AXIS2_PLACEMENT_3D ( 'NONE', #22934, #17722, #3142 ) ;
#19476=AXIS2_PLACEMENT_3D ( 'NONE', #24175, #4536, #16890 ) ;
#19502=EDGE_CURVE ( 'NONE', #19797, #23537, #13290, .T. ) ;
#19518=DIRECTION ( 'NONE',  ( -1.000000000000000000, -3.053848253006669023E-16, 2.042510438544995415E-16 ) ) ;
#19526=VECTOR ( 'NONE', #12402, 1000.000000000000000 ) ;
#19529=ORIENTED_EDGE ( 'NONE', *, *, #2101, .T. ) ;
#19539=CARTESIAN_POINT ( 'NONE',  ( -61.39879105983192886, -2.652949782970507098, 0.5017753628371410812 ) ) ;
#19545=EDGE_CURVE ( 'NONE', #7685, #4534, #29664, .T. ) ;
#19550=DIRECTION ( 'NONE',  ( 0.000000000000000000, -0.9996898646859343485, -0.02490330187381124133 ) ) ;
#19563=CARTESIAN_POINT ( 'NONE',  ( -60.59999999999997300, -2.464733277392923139, 0.9389111926722781831 ) ) ;
#19575=DIRECTION ( 'NONE',  ( 0.000000000000000000, 0.9996898646859344595, 0.02490330187381124133 ) ) ;
#19592=EDGE_CURVE ( 'NONE', #20831, #22178, #9530, .T. ) ;
#19598=CIRCLE ( 'NONE', #5418, 1.613789466889706814 ) ;
#19663=CARTESIAN_POINT ( 'NONE',  ( -60.49999999999997868, 1.656632322739229403E-15, 1.870925083934595927E-15 ) ) ;
#19689=CARTESIAN_POINT ( 'NONE',  ( -62.09999999999997300, -2.643914563970546805, -0.2822557264641659680 ) ) ;
#19690=VERTEX_POINT ( 'NONE', #21256 ) ;
#19692=PLANE ( 'NONE',  #23949 ) ;
#19712=CARTESIAN_POINT ( 'NONE',  ( -73.89999999999997726, 0.4598573377555274511, 0.01145551886195783631 ) ) ;
#19728=CYLINDRICAL_SURFACE ( 'NONE', #14976, 2.625000000000000444 ) ;
#19761=ORIENTED_EDGE ( 'NONE', *, *, #3780, .F. ) ;
#19762=DIRECTION ( 'NONE',  ( 0.000000000000000000, -0.9996898646859344595, -0.02490330187381124827 ) ) ;
#19765=ORIENTED_EDGE ( 'NONE', *, *, #27270, .T. ) ;
#19783=CARTESIAN_POINT ( 'NONE',  ( -67.89999999999997726, 1.599503783497494780, 0.03984528299810137508 ) ) ;
#19797=VERTEX_POINT ( 'NONE', #30673 ) ;
#19800=CARTESIAN_POINT ( 'NONE',  ( -73.85208152723558328, -2.420890761855879333E-15, 4.598101673502850081E-15 ) ) ;
#19801=DIRECTION ( 'NONE',  ( 1.000000000000000000, 3.053848253006669023E-16, -2.042510438544995415E-16 ) ) ;
#19830=CARTESIAN_POINT ( 'NONE',  ( -62.08976859767152234, -2.518353679445345605, 0.1831464729044566531 ) ) ;
#19832=LINE ( 'NONE', #29620, #8396 ) ;
#19840=CARTESIAN_POINT ( 'NONE',  ( -61.39959699979583263, -2.652859410556386521, 0.5023315908532165475 ) ) ;
#19846=ORIENTED_EDGE ( 'NONE', *, *, #19294, .F. ) ;
#19859=( BOUNDED_CURVE ( )  B_SPLINE_CURVE ( 3, ( #24777, #3086, #8002, #17665 ),
 .UNSPECIFIED., .F., .T. ) 
 B_SPLINE_CURVE_WITH_KNOTS ( ( 4, 4 ),
 ( 1.164632096430649133, 1.274397363402604677 ),
 .UNSPECIFIED. ) 
 CURVE ( )  GEOMETRIC_REPRESENTATION_ITEM ( )  RATIONAL_B_SPLINE_CURVE ( ( 1.000000000000000000, 0.9989962175098910935, 0.9989962175098910935, 1.000000000000000000 ) ) 
 REPRESENTATION_ITEM ( '' )  );
#19868=CARTESIAN_POINT ( 'NONE',  ( -61.34999999999997300, -2.435425537339440449, 0.6665789166144534539 ) ) ;
#19885=CARTESIAN_POINT ( 'NONE',  ( -63.86464466094066239, 6.291209007590390943E-16, 2.558157268131197822E-15 ) ) ;
#19909=CARTESIAN_POINT ( 'NONE',  ( -61.34999999999997300, -2.580661732147724319, -0.5877664123773247429 ) ) ;
#19921=ORIENTED_EDGE ( 'NONE', *, *, #16715, .T. ) ;
#19926=CARTESIAN_POINT ( 'NONE',  ( -60.59999999999998010, -2.414926673651788924, -1.060468536699751940 ) ) ;
#19939=CARTESIAN_POINT ( 'NONE',  ( -60.60558231549867969, -2.497277651495709794, 0.9543206905132385343 ) ) ;
#19955=VERTEX_POINT ( 'NONE', #15107 ) ;
#19969=VECTOR ( 'NONE', #25677, 999.9999999999998863 ) ;
#20020=VECTOR ( 'NONE', #30202, 1000.000000000000000 ) ;
#20044=EDGE_LOOP ( 'NONE', ( #16575, #30421, #9181, #31019, #30864, #19363, #18652, #26700, #21004 ) ) ;
#20060=ADVANCED_FACE ( 'NONE', ( #30767 ), #15944, .T. ) ;
#20069=TOROIDAL_SURFACE ( 'NONE', #21592, 1.260000000000000009, 0.01000000000000000021 ) ;
#20108=ADVANCED_FACE ( 'NONE', ( #9076 ), #1618, .T. ) ;
#20120=EDGE_LOOP ( 'NONE', ( #24034, #15503, #28605, #13851, #6414, #24283 ) ) ;
#20132=DIRECTION ( 'NONE',  ( -1.000000000000000000, -3.053848253006669023E-16, 2.042510438544995415E-16 ) ) ;
#20133=EDGE_LOOP ( 'NONE', ( #5265, #17627 ) ) ;
#20152=CARTESIAN_POINT ( 'NONE',  ( -61.39999999999998437, -2.652806974455509170, 0.5026083527760007996 ) ) ;
#20155=CARTESIAN_POINT ( 'NONE',  ( -62.07235880193731248, -2.517270094365763100, 0.1974334673667717810 ) ) ;
#20156=CARTESIAN_POINT ( 'NONE',  ( -64.32138495697122949, 4.896393452479652361E-16, 2.651446950365857792E-15 ) ) ;
#20158=CARTESIAN_POINT ( 'NONE',  ( -62.09999999999997300, -2.717421493829955459, -0.3515446183602667918 ) ) ;
#20161=CARTESIAN_POINT ( 'NONE',  ( -67.88621053311027254, -5.990042905486032463E-16, 3.379566295451473069E-15 ) ) ;
#20164=LINE ( 'NONE', #10943, #28183 ) ;
#20167=CARTESIAN_POINT ( 'NONE',  ( -62.34999999999997300, 1.091670395932995432E-15, 2.248789515065420326E-15 ) ) ;
#20204=CIRCLE ( 'NONE', #20728, 1.351996603031850208 ) ;
#20254=CARTESIAN_POINT ( 'NONE',  ( -73.89999999999997726, -2.435524336289708093E-15, 4.607889071584891164E-15 ) ) ;
#20263=DIRECTION ( 'NONE',  ( 0.7071067811865462405, 0.7068874824028876791, 0.01760929362890746239 ) ) ;
#20266=EDGE_CURVE ( 'NONE', #8829, #13929, #14925, .T. ) ;
#20278=ORIENTED_EDGE ( 'NONE', *, *, #14263, .T. ) ;
#20282=CARTESIAN_POINT ( 'NONE',  ( -67.33025350686975230, 2.149980434289362030, 0.05355822207392273160 ) ) ;
#20299=EDGE_CURVE ( 'NONE', #5910, #14916, #17298, .T. ) ;
#20301=DIRECTION ( 'NONE',  ( 0.000000000000000000, -0.9996898646859344595, -0.02490330187381124133 ) ) ;
#20322=CARTESIAN_POINT ( 'NONE',  ( -60.60807700862574166, -2.449477319984247892, -1.080610302189543459 ) ) ;
#20326=VERTEX_POINT ( 'NONE', #7326 ) ;
#20334=ORIENTED_EDGE ( 'NONE', *, *, #19592, .F. ) ;
#20357=ADVANCED_FACE ( 'NONE', ( #22513 ), #10780, .T. ) ;
#20363=CARTESIAN_POINT ( 'NONE',  ( -62.07342829042941901, -2.504415692620788114, -0.3217612745991157430 ) ) ;
#20366=CARTESIAN_POINT ( 'NONE',  ( -61.39639585615719142, -2.605025371766806153, 0.7093239484020297247 ) ) ;
#20372=VERTEX_POINT ( 'NONE', #17920 ) ;
#20383=CARTESIAN_POINT ( 'NONE',  ( -60.85363833753317664, -2.496020359703504443, 0.8457863545849919618 ) ) ;
#20419=CARTESIAN_POINT ( 'NONE',  ( -60.64999999999998437, -2.511038422848939078, 0.9923134781793048198 ) ) ;
#20444=CARTESIAN_POINT ( 'NONE',  ( -61.39263535326296051, -2.625539631637058502, -0.6290288465273202734 ) ) ;
#20446=ORIENTED_EDGE ( 'NONE', *, *, #6548, .T. ) ;
#20469=EDGE_CURVE ( 'NONE', #24563, #29552, #20626, .T. ) ;
#20473=CARTESIAN_POINT ( 'NONE',  ( -60.60075002049966031, -2.435642456719447679, -1.068919490937977113 ) ) ;
#20486=ORIENTED_EDGE ( 'NONE', *, *, #13713, .F. ) ;
#20494=FACE_OUTER_BOUND ( 'NONE', #21990, .T. ) ;
#20499=CARTESIAN_POINT ( 'NONE',  ( -64.29999999999996874, 4.961699865966959239E-16, 2.647079050581693988E-15 ) ) ;
#20515=ORIENTED_EDGE ( 'NONE', *, *, #5877, .T. ) ;
#20516=VERTEX_POINT ( 'NONE', #1735 ) ;
#20534=EDGE_CURVE ( 'NONE', #2594, #6393, #28986, .T. ) ;
#20543=EDGE_LOOP ( 'NONE', ( #21415, #26194, #7027, #25896 ) ) ;
#20551=ORIENTED_EDGE ( 'NONE', *, *, #5530, .T. ) ;
#20558=CARTESIAN_POINT ( 'NONE',  ( -61.34999999999997300, -2.515554072771550853, -0.7899129066418597578 ) ) ;
#20572=CIRCLE ( 'NONE', #10446, 1.302039949377232331 ) ;
#20575=EDGE_CURVE ( 'NONE', #14583, #3014, #2192, .T. ) ;
#20578=CARTESIAN_POINT ( 'NONE',  ( -60.59999999999997300, -2.481395594095113122, 0.9440358133373861760 ) ) ;
#20589=AXIS2_PLACEMENT_3D ( 'NONE', #8858, #18550, #21255 ) ;
#20592=CARTESIAN_POINT ( 'NONE',  ( -60.64999999999998437, 1.610824598944129570E-15, 1.901562740512771401E-15 ) ) ;
#20626=LINE ( 'NONE', #4274, #17872 ) ;
#20634=CARTESIAN_POINT ( 'NONE',  ( -60.60214168571716442, -2.439458054579491719, -1.071672411231956223 ) ) ;
#20643=SURFACE_STYLE_USAGE ( .BOTH. , #8577 ) ;
#20675=CARTESIAN_POINT ( 'NONE',  ( -61.39919102937896156, -2.604635884043592586, 0.7112281530754581693 ) ) ;
#20677=ADVANCED_FACE ( 'NONE', ( #24525 ), #17884, .F. ) ;
#20699=CARTESIAN_POINT ( 'NONE',  ( -60.87073935753531373, -2.544307234692274378, 0.9096008698628265110 ) ) ;
#20728=AXIS2_PLACEMENT_3D ( 'NONE', #19800, #29434, #169 ) ;
#20748=EDGE_CURVE ( 'NONE', #20372, #2467, #19411, .T. ) ;
#20760=AXIS2_PLACEMENT_3D ( 'NONE', #3712, #30790, #16381 ) ;
#20768=VECTOR ( 'NONE', #18924, 1000.000000000000000 ) ;
#20774=CARTESIAN_POINT ( 'NONE',  ( -62.09999999999997300, -2.692057237979972317, -0.3088123856379243470 ) ) ;
#20776=CARTESIAN_POINT ( 'NONE',  ( -62.06507697720029171, -2.652888718249335032, -0.3385697102886689458 ) ) ;
#20820=ORIENTED_EDGE ( 'NONE', *, *, #15478, .T. ) ;
#20831=VERTEX_POINT ( 'NONE', #10278 ) ;
#20877=CIRCLE ( 'NONE', #1194, 2.700000000000000178 ) ;
#20896=DIRECTION ( 'NONE',  ( 0.000000000000000000, 0.9996898646859343485, 0.02490330187381124133 ) ) ;
#20935=VERTEX_POINT ( 'NONE', #16915 ) ;
#20938=FILL_AREA_STYLE ('',( #13470 ) ) ;
#20955=AXIS2_PLACEMENT_3D ( 'NONE', #28812, #16782, #4723 ) ;
#20982=EDGE_CURVE ( 'NONE', #22436, #24250, #1172, .T. ) ;
#20986=DIRECTION ( 'NONE',  ( -1.000000000000000000, -3.053848253006669023E-16, 2.042510438544995415E-16 ) ) ;
#21004=ORIENTED_EDGE ( 'NONE', *, *, #5279, .T. ) ;
#21018=DIRECTION ( 'NONE',  ( 3.002035892788117459E-16, -0.9996898646859343485, -0.02490330187381123786 ) ) ;
#21049=VERTEX_POINT ( 'NONE', #27188 ) ;
#21068=AXIS2_PLACEMENT_3D ( 'NONE', #27592, #3388, #22718 ) ;
#21070=CARTESIAN_POINT ( 'NONE',  ( -61.34999999999997300, -2.565134197206211386, 0.6652717868084008224 ) ) ;
#21123=VECTOR ( 'NONE', #21250, 999.9999999999998863 ) ;
#21132=DIRECTION ( 'NONE',  ( -0.9396926207859088720, -0.008517430876163569961, 0.3419140708011006446 ) ) ;
#21138=VERTEX_POINT ( 'NONE', #2968 ) ;
#21163=DIRECTION ( 'NONE',  ( 1.000000000000000000, 3.053848253006669023E-16, -2.042510438544995415E-16 ) ) ;
#21179=ORIENTED_EDGE ( 'NONE', *, *, #11797, .F. ) ;
#21190=EDGE_LOOP ( 'NONE', ( #1704, #22242, #22523, #1659, #25323, #24629, #7113 ) ) ;
#21213=ORIENTED_EDGE ( 'NONE', *, *, #7165, .F. ) ;
#21247=DIRECTION ( 'NONE',  ( -1.000000000000000000, -3.053848253006669023E-16, 2.042510438544995415E-16 ) ) ;
#21250=DIRECTION ( 'NONE',  ( -3.002035892788117459E-16, 0.9996898646859344595, 0.02490330187381124133 ) ) ;
#21255=DIRECTION ( 'NONE',  ( 0.000000000000000000, 0.9996898646859343485, 0.02490330187381123439 ) ) ;
#21256=CARTESIAN_POINT ( 'NONE',  ( -62.09999999999997300, -2.749147127886318653, -0.06848408015297871576 ) ) ;
#21258=DIRECTION ( 'NONE',  ( -3.002035892788117459E-16, 0.9996898646859344595, 0.02490330187381124133 ) ) ;
#21301=CARTESIAN_POINT ( 'NONE',  ( -61.34999999999997300, -2.614490477541997926, 0.4599799668244957118 ) ) ;
#21311=ORIENTED_EDGE ( 'NONE', *, *, #25422, .T. ) ;
#21314=ORIENTED_EDGE ( 'NONE', *, *, #24978, .T. ) ;
#21321=CARTESIAN_POINT ( 'NONE',  ( -62.09999999999997300, -2.729900678946055148, 0.2118983792693960311 ) ) ;
#21367=EDGE_CURVE ( 'NONE', #4534, #7685, #15866, .T. ) ;
#21379=ORIENTED_EDGE ( 'NONE', *, *, #27672, .F. ) ;
#21399=EDGE_CURVE ( 'NONE', #28721, #22270, #1321, .T. ) ;
#21411=ORIENTED_EDGE ( 'NONE', *, *, #5441, .F. ) ;
#21415=ORIENTED_EDGE ( 'NONE', *, *, #24099, .F. ) ;
#21437=CARTESIAN_POINT ( 'NONE',  ( -73.89999999999997726, -1.349581317326014052, -0.03361945752964041328 ) ) ;
#21452=ORIENTED_EDGE ( 'NONE', *, *, #14514, .F. ) ;
#21469=ORIENTED_EDGE ( 'NONE', *, *, #16270, .T. ) ;
#21470=CARTESIAN_POINT ( 'NONE',  ( -61.14517784068949879, -2.578482729018109598, 0.8069458425966854476 ) ) ;
#21530=DIRECTION ( 'NONE',  ( -3.002035892788116966E-16, 0.9996898646859343485, 0.02490330187381124133 ) ) ;
#21539=AXIS2_PLACEMENT_3D ( 'NONE', #4009, #13797, #23335 ) ;
#21540=CARTESIAN_POINT ( 'NONE',  ( -61.36728013402707660, -2.617907752630248108, -0.6089896480292835701 ) ) ;
#21554=CARTESIAN_POINT ( 'NONE',  ( -62.14999999999998437, 1.152747360993128871E-15, 2.207939306294521009E-15 ) ) ;
#21585=TOROIDAL_SURFACE ( 'NONE', #14971, 2.750000000000000444, 0.05000000000000000278 ) ;
#21592=AXIS2_PLACEMENT_3D ( 'NONE', #6587, #3725, #18468 ) ;
#21595=CONICAL_SURFACE ( 'NONE', #16000, 2.150000000000000355, 0.03277514440407566787 ) ;
#21639=CIRCLE ( 'NONE', #3879, 2.249352573995730520 ) ;
#21643=ADVANCED_FACE ( 'NONE', ( #5224 ), #1699, .T. ) ;
#21662=AXIS2_PLACEMENT_3D ( 'NONE', #7118, #18684, #25946 ) ;
#21669=AXIS2_PLACEMENT_3D ( 'NONE', #10137, #19801, #29435 ) ;
#21697=CARTESIAN_POINT ( 'NONE',  ( -61.60258317630325564, -2.642987027397695865, -0.5593832590402626481 ) ) ;
#21710=CARTESIAN_POINT ( 'NONE',  ( -62.09999999999997300, 1.168016602258162478E-15, 2.197726754101795588E-15 ) ) ;
#21717=CARTESIAN_POINT ( 'NONE',  ( -62.06277111861474793, -2.675496248757341267, 0.2149375022555932713 ) ) ;
#21718=CARTESIAN_POINT ( 'NONE',  ( -61.57740687343568453, -2.676030259482950591, 0.3736822453871994631 ) ) ;
#21746=AXIS2_PLACEMENT_3D ( 'NONE', #18522, #2187, #16300 ) ;
#21799=AXIS2_PLACEMENT_3D ( 'NONE', #9879, #12251, #17021 ) ;
#21812=VERTEX_POINT ( 'NONE', #18058 ) ;
#21834=ADVANCED_FACE ( 'NONE', ( #27702 ), #15041, .T. ) ;
#21839=ADVANCED_FACE ( 'NONE', ( #24698, #782 ), #3012, .T. ) ;
#21844=ORIENTED_EDGE ( 'NONE', *, *, #22321, .F. ) ;
#21892=EDGE_LOOP ( 'NONE', ( #12355, #11939 ) ) ;
#21899=ORIENTED_EDGE ( 'NONE', *, *, #14716, .T. ) ;
#21908=CARTESIAN_POINT ( 'NONE',  ( -61.39959552429773026, -2.565909676969820641, -0.8403020935398156643 ) ) ;
#21909=( BOUNDED_SURFACE ( )  B_SPLINE_SURFACE ( 3, 2, ( 
 ( #9353, #14399, #16651 ),
 ( #4120, #9034, #26292 ),
 ( #23443, #18708, #2213 ),
 ( #4594, #28352, #9528 ) ),
 .UNSPECIFIED., .F., .F., .T. ) 
 B_SPLINE_SURFACE_WITH_KNOTS ( ( 4, 4 ),
 ( 3, 3 ),
 ( 3.756617526051016459E-05, 0.0002104436212403357762 ),
 ( 0.000000000000000000, 1.000000000000000000 ),
 .UNSPECIFIED. ) 
 GEOMETRIC_REPRESENTATION_ITEM ( )  RATIONAL_B_SPLINE_SURFACE ( (
 ( 1.000000000000000000, 0.7071067811865965336, 1.000000000000000000),
 ( 1.000000000000000000, 0.7737094907949337852, 1.000000000000000000),
 ( 1.000000000000000000, 0.8271097373158977639, 1.000000000000000000),
 ( 1.000000000000000000, 0.8191520442890480869, 1.000000000000000000) ) ) 
 REPRESENTATION_ITEM ( '' )  SURFACE ( )  );
#21948=DIRECTION ( 'NONE',  ( 1.000000000000000000, 3.053848253006669023E-16, -2.042510438544995415E-16 ) ) ;
#21955=CARTESIAN_POINT ( 'NONE',  ( -74.39999999999997726, -2.588216748940040213E-15, 4.710014593512140639E-15 ) ) ;
#21990=EDGE_LOOP ( 'NONE', ( #15152, #17491, #9127, #9829 ) ) ;
#22013=TOROIDAL_SURFACE ( 'NONE', #18969, 2.750000000000000000, 0.05000000000000000278 ) ;
#22038=CARTESIAN_POINT ( 'NONE',  ( -61.34999999999997300, -2.609922480197373940, 0.4591346723570145505 ) ) ;
#22075=ORIENTED_EDGE ( 'NONE', *, *, #10025, .F. ) ;
#22083=DIRECTION ( 'NONE',  ( -1.000000000000000000, -3.053848253006669023E-16, 2.042510438544995415E-16 ) ) ;
#22103=CONICAL_SURFACE ( 'NONE', #20589, 2.250000000000000444, 0.7853981633974536081 ) ;
#22116=ORIENTED_EDGE ( 'NONE', *, *, #20469, .T. ) ;
#22118=DIRECTION ( 'NONE',  ( 1.000000000000000000, 3.053848253006669023E-16, -2.042510438544995415E-16 ) ) ;
#22124=CIRCLE ( 'NONE', #16557, 0.4600000000000000755 ) ;
#22127=EDGE_CURVE ( 'NONE', #20935, #11715, #2737, .T. ) ;
#22134=AXIS2_PLACEMENT_3D ( 'NONE', #12469, #17553, #12936 ) ;
#22138=ORIENTED_EDGE ( 'NONE', *, *, #25086, .F. ) ;
#22170=VECTOR ( 'NONE', #28359, 1000.000000000000114 ) ;
#22178=VERTEX_POINT ( 'NONE', #31167 ) ;
#22208=COLOUR_RGB ( '', 0.08235294, 0.09019608, 0.10196078) ;
#22212=CARTESIAN_POINT ( 'NONE',  ( -61.39266396720692143, -2.567250461644490223, -0.8356799977092136400 ) ) ;
#22218=ORIENTED_EDGE ( 'NONE', *, *, #30793, .T. ) ;
#22227=ORIENTED_EDGE ( 'NONE', *, *, #1253, .T. ) ;
#22230=CARTESIAN_POINT ( 'NONE',  ( -61.39999999999998437, -2.604492677689918878, 0.7117709546332967596 ) ) ;
#22242=ORIENTED_EDGE ( 'NONE', *, *, #12895, .T. ) ;
#22251=DIRECTION ( 'NONE',  ( 1.000000000000000000, 3.053848253006669023E-16, -2.042510438544995415E-16 ) ) ;
#22252=AXIS2_PLACEMENT_3D ( 'NONE', #12972, #15517, #29916 ) ;
#22260=CARTESIAN_POINT ( 'NONE',  ( -63.86464466094066239, 6.291209007590390943E-16, 2.558157268131197822E-15 ) ) ;
#22270=VERTEX_POINT ( 'NONE', #17705 ) ;
#22274=CIRCLE ( 'NONE', #20760, 2.525000000000001243 ) ;
#22294=CARTESIAN_POINT ( 'NONE',  ( -67.32861504302871936, -4.287230892216076523E-16, 3.265676834553754426E-15 ) ) ;
#22315=LINE ( 'NONE', #17720, #27097 ) ;
#22321=EDGE_CURVE ( 'NONE', #28152, #1827, #22496, .T. ) ;
#22324=DIRECTION ( 'NONE',  ( -1.000000000000000000, -3.053848253006669023E-16, 2.042510438544995415E-16 ) ) ;
#22351=CARTESIAN_POINT ( 'NONE',  ( -60.64999999999998437, 1.610824598944129570E-15, 1.901562740512771401E-15 ) ) ;
#22358=CARTESIAN_POINT ( 'NONE',  ( -61.38069258722538279, -2.566273914340431173, -0.8266263692889775916 ) ) ;
#22364=EDGE_CURVE ( 'NONE', #1635, #20831, #7328, .T. ) ;
#22372=CARTESIAN_POINT ( 'NONE',  ( -60.63660384741033482, -2.460988642455861797, -1.107171701358785620 ) ) ;
#22373=EDGE_LOOP ( 'NONE', ( #2647, #7567, #21379, #24752 ) ) ;
#22387=EDGE_CURVE ( 'NONE', #11253, #14068, #6301, .T. ) ;
#22424=EDGE_CURVE ( 'NONE', #7997, #66, #22995, .T. ) ;
#22433=CIRCLE ( 'NONE', #14818, 1.613789466889706814 ) ;
#22436=VERTEX_POINT ( 'NONE', #3599 ) ;
#22444=DIRECTION ( 'NONE',  ( 0.000000000000000000, 0.9996898646859344595, 0.02490330187381124827 ) ) ;
#22467=CIRCLE ( 'NONE', #20955, 0.05000000000000012074 ) ;
#22468=CARTESIAN_POINT ( 'NONE',  ( -60.60214168571716442, -2.489792084731451194, 0.9488797246527581608 ) ) ;
#22477=UNCERTAINTY_MEASURE_WITH_UNIT (LENGTH_MEASURE( 1.000000000000000082E-05 ), #9070, 'distance_accuracy_value', 'NONE');
#22496=CIRCLE ( 'NONE', #11870, 2.263970382088065225 ) ;
#22498=EDGE_CURVE ( 'NONE', #3131, #29448, #254, .T. ) ;
#22508=CARTESIAN_POINT ( 'NONE',  ( -62.07735545010103806, -2.517494014746469499, 0.1945804328892600521 ) ) ;
#22513=FACE_OUTER_BOUND ( 'NONE', #14495, .T. ) ;
#22520=CARTESIAN_POINT ( 'NONE',  ( -61.35192115139415137, -2.623188642970683215, 0.4629488832698942513 ) ) ;
#22523=ORIENTED_EDGE ( 'NONE', *, *, #17070, .T. ) ;
#22567=CARTESIAN_POINT ( 'NONE',  ( -73.85208152723558328, 1.351577301140750587, 0.03366917953767410016 ) ) ;
#22576=ORIENTED_EDGE ( 'NONE', *, *, #27010, .F. ) ;
#22580=VERTEX_POINT ( 'NONE', #23861 ) ;
#22592=DIRECTION ( 'NONE',  ( 0.000000000000000000, -0.9996898646859346815, -0.02490330187379791865 ) ) ;
#22595=CARTESIAN_POINT ( 'NONE',  ( -60.58528264635175731, -2.531045389859400974, 0.9426176302699454945 ) ) ;
#22598=VECTOR ( 'NONE', #10701, 1000.000000000000000 ) ;
#22611=ADVANCED_FACE ( 'NONE', ( #29229 ), #27019, .T. ) ;
#22667=AXIS2_PLACEMENT_3D ( 'NONE', #20499, #15735, #28063 ) ;
#22686=CARTESIAN_POINT ( 'NONE',  ( -62.06710100716625789, -2.694091267595633887, 0.1949429447076614641 ) ) ;
#22688=CARTESIAN_POINT ( 'NONE',  ( -62.09999999999997300, -2.712886303669590049, -0.3394508044491614807 ) ) ;
#22690=DIRECTION ( 'NONE',  ( 0.000000000000000000, 0.9996898646859344595, 0.02490330187381124133 ) ) ;
#22697=CARTESIAN_POINT ( 'NONE',  ( -60.59999999999997300, -2.426837276046140079, -1.064406330116907329 ) ) ;
#22718=DIRECTION ( 'NONE',  ( 0.000000000000000000, -0.9996898646859344595, -0.02490330187381124133 ) ) ;
#22729=DIRECTION ( 'NONE',  ( 1.000000000000000000, 3.053848253006669023E-16, -2.042510438544995415E-16 ) ) ;
#22747=AXIS2_PLACEMENT_3D ( 'NONE', #19663, #17272, #2110 ) ;
#22758=CARTESIAN_POINT ( 'NONE',  ( -61.40479058095097287, -2.604980992110456306, 0.7099817115554608593 ) ) ;
#22779=CIRCLE ( 'NONE', #28321, 0.04999999999999988481 ) ;
#22790=CARTESIAN_POINT ( 'NONE',  ( -61.34999999999997300, 1.397055221233662433E-15, 2.044538471210920981E-15 ) ) ;
#22808=DIRECTION ( 'NONE',  ( 0.000000000000000000, 0.9996898646859344595, 0.02490330187381119623 ) ) ;
#22822=DIRECTION ( 'NONE',  ( 2.117927888850091331E-16, -0.02490330187381135929, 0.9996898646859343485 ) ) ;
#22828=DIRECTION ( 'NONE',  ( -1.000000000000000000, -3.053848253006669023E-16, 2.042510438544995415E-16 ) ) ;
#22847=CARTESIAN_POINT ( 'NONE',  ( -60.61073679674431958, -2.452477434632136077, -1.083948463035139476 ) ) ;
#22863=TOROIDAL_SURFACE ( 'NONE', #29390, 1.302039949377232331, 0.05000000000000000278 ) ;
#22876=ORIENTED_EDGE ( 'NONE', *, *, #20266, .T. ) ;
#22881=CARTESIAN_POINT ( 'NONE',  ( -62.09999999999997300, -2.509696570289218442, -0.2775754403374581791 ) ) ;
#22884=CARTESIAN_POINT ( 'NONE',  ( -61.37479624186750016, -2.602756195442594844, 0.6931813454126620755 ) ) ;
#22908=( BOUNDED_CURVE ( )  B_SPLINE_CURVE ( 3, ( #26797, #30084, #11092, #3511 ),
 .UNSPECIFIED., .F., .T. ) 
 B_SPLINE_CURVE_WITH_KNOTS ( ( 4, 4 ),
 ( 5.008787943776981777, 5.118553210748935989 ),
 .UNSPECIFIED. ) 
 CURVE ( )  GEOMETRIC_REPRESENTATION_ITEM ( )  RATIONAL_B_SPLINE_CURVE ( ( 1.000000000000000000, 0.9989962175098912045, 0.9989962175098912045, 1.000000000000000000 ) ) 
 REPRESENTATION_ITEM ( '' )  );
#22922=EDGE_CURVE ( 'NONE', #66, #7997, #6826, .T. ) ;
#22930=DIRECTION ( 'NONE',  ( 1.000000000000000000, 3.053848253006669023E-16, -2.042510438544995415E-16 ) ) ;
#22934=CARTESIAN_POINT ( 'NONE',  ( -62.04999999999998295, -2.692921195145432822, 0.1479728852616695456 ) ) ;
#22937=EDGE_CURVE ( 'NONE', #28072, #1808, #11384, .T. ) ;
#22940=CARTESIAN_POINT ( 'NONE',  ( -60.59999999999997300, -2.476825173781434852, 0.9422510591782664591 ) ) ;
#22959=PLANE ( 'NONE',  #11484 ) ;
#22995=CIRCLE ( 'NONE', #4264, 0.4600000000000000755 ) ;
#23007=ORIENTED_EDGE ( 'NONE', *, *, #25476, .T. ) ;
#23064=VECTOR ( 'NONE', #5527, 1000.000000000000000 ) ;
#23094=FACE_OUTER_BOUND ( 'NONE', #11691, .T. ) ;
#23124=COLOUR_RGB ( '', 0.08235294, 0.09019608, 0.10196078) ;
#23126=EDGE_LOOP ( 'NONE', ( #2509, #25626, #2898, #27701 ) ) ;
#23170=AXIS2_PLACEMENT_3D ( 'NONE', #12277, #11980, #14804 ) ;
#23174=ORIENTED_EDGE ( 'NONE', *, *, #20982, .T. ) ;
#23182=CIRCLE ( 'NONE', #15065, 0.04999999999999988481 ) ;
#23200=EDGE_LOOP ( 'NONE', ( #4202, #16760, #8038, #28449 ) ) ;
#23215=DIRECTION ( 'NONE',  ( -1.000000000000000000, -3.053848253006669023E-16, 2.042510438544995415E-16 ) ) ;
#23217=CARTESIAN_POINT ( 'NONE',  ( -60.49999999999997868, 2.524216908331986975, 0.06288083723137545544 ) ) ;
#23219=CARTESIAN_POINT ( 'NONE',  ( -61.38768957378469793, -2.555570530917468997, 0.6498638426362197684 ) ) ;
#23253=EDGE_CURVE ( 'NONE', #2488, #20831, #20877, .T. ) ;
#23278=VERTEX_POINT ( 'NONE', #29272 ) ;
#23286=CARTESIAN_POINT ( 'NONE',  ( -60.89492752328840908, -2.499300970757945439, -1.026269669383801153 ) ) ;
#23296=LINE ( 'NONE', #8854, #18498 ) ;
#23301=CARTESIAN_POINT ( 'NONE',  ( -62.06722781964786151, -2.633694437091016027, -0.3282923398133328896 ) ) ;
#23335=DIRECTION ( 'NONE',  ( 3.002035892788117459E-16, -0.9996898646859343485, -0.02490330187381124133 ) ) ;
#23342=ORIENTED_EDGE ( 'NONE', *, *, #8474, .F. ) ;
#23362=FACE_OUTER_BOUND ( 'NONE', #16189, .T. ) ;
#23388=DIRECTION ( 'NONE',  ( 0.000000000000000000, -0.9996898646859344595, -0.02490330187381124480 ) ) ;
#23443=CARTESIAN_POINT ( 'NONE',  ( -62.09999999999998010, -2.687742116683883520, -0.2820114153134715140 ) ) ;
#23444=DIRECTION ( 'NONE',  ( -2.117927888850090838E-16, 0.02490330187381123786, -0.9996898646859343485 ) ) ;
#23447=ORIENTED_EDGE ( 'NONE', *, *, #13638, .T. ) ;
#23449=DIRECTION ( 'NONE',  ( 0.000000000000000000, 0.9996898646859344595, 0.02490330187381124133 ) ) ;
#23456=EDGE_LOOP ( 'NONE', ( #10707, #2073, #28155, #30514 ) ) ;
#23465=VERTEX_POINT ( 'NONE', #28109 ) ;
#23477=DIRECTION ( 'NONE',  ( 0.9991330730923518866, -0.04161763361012198875, -0.001036738022138846901 ) ) ;
#23493=ORIENTED_EDGE ( 'NONE', *, *, #7165, .T. ) ;
#23497=EDGE_CURVE ( 'NONE', #24203, #1635, #23906, .T. ) ;
#23500=DIRECTION ( 'NONE',  ( 0.000000000000000000, -0.9996898646859343485, -0.02490330187381143562 ) ) ;
#23506=FACE_OUTER_BOUND ( 'NONE', #24466, .T. ) ;
#23537=VERTEX_POINT ( 'NONE', #12264 ) ;
#23590=SHAPE_DEFINITION_REPRESENTATION ( #7112, #29923 ) ;
#23597=FACE_OUTER_BOUND ( 'NONE', #22373, .T. ) ;
#23611=AXIS2_PLACEMENT_3D ( 'NONE', #26173, #7488, #5101 ) ;
#23646=CIRCLE ( 'NONE', #3924, 2.136029617911934686 ) ;
#23669=DIRECTION ( 'NONE',  ( 1.000000000000000000, 3.053848253006669023E-16, -2.042510438544995415E-16 ) ) ;
#23672=ORIENTED_EDGE ( 'NONE', *, *, #22424, .F. ) ;
#23679=DIRECTION ( 'NONE',  ( 2.466396912850936180E-16, -0.1459676528264960971, 0.9892893632948469573 ) ) ;
#23687=VECTOR ( 'NONE', #28512, 999.9999999999998863 ) ;
#23722=CARTESIAN_POINT ( 'NONE',  ( -61.34999999999997300, -2.635021238245644160, -0.5887810068220489246 ) ) ;
#23767=DIRECTION ( 'NONE',  ( 0.000000000000000000, -0.9996898646859344595, -0.02490330187381105745 ) ) ;
#23772=CIRCLE ( 'NONE', #7577, 2.650000000000000799 ) ;
#23777=CARTESIAN_POINT ( 'NONE',  ( -60.59999999999997300, 1.626093840209163176E-15, 1.891350188320046374E-15 ) ) ;
#23782=ORIENTED_EDGE ( 'NONE', *, *, #31068, .F. ) ;
#23785=( BOUNDED_SURFACE ( )  B_SPLINE_SURFACE ( 3, 2, ( 
 ( #29708, #27333, #14245 ),
 ( #23916, #21718, #2209 ),
 ( #11874, #5644, #31196 ),
 ( #9675, #4903, #15297 ) ),
 .UNSPECIFIED., .F., .F., .F. ) 
 B_SPLINE_SURFACE_WITH_KNOTS ( ( 4, 4 ),
 ( 3, 3 ),
 ( 1.353422612224536969, 1.454597276681381723 ),
 ( 0.000000000000000000, 1.000000000000000000 ),
 .UNSPECIFIED. ) 
 GEOMETRIC_REPRESENTATION_ITEM ( )  RATIONAL_B_SPLINE_SURFACE ( (
 ( 1.000000000000000000, 0.6314033403188393789, 1.000000000000000000),
 ( 1.000000000000000000, 0.6436559554927198112, 1.000000000000000000),
 ( 1.000000000000000000, 0.6556885524390240194, 1.000000000000000000),
 ( 1.000000000000000000, 0.6674781514195016197, 1.000000000000000000) ) ) 
 REPRESENTATION_ITEM ( '' )  SURFACE ( )  );
#23806=LINE ( 'NONE', #21437, #13954 ) ;
#23815=ADVANCED_FACE ( 'NONE', ( #27926 ), #27441, .F. ) ;
#23831=CARTESIAN_POINT ( 'NONE',  ( -60.59999999999998010, -2.292917048100124866, -1.057429151542457868 ) ) ;
#23838=CARTESIAN_POINT ( 'NONE',  ( -62.09999999999997300, -2.724924404790626031, 0.2013854104211484086 ) ) ;
#23841=CARTESIAN_POINT ( 'NONE',  ( -60.64999999999998437, -2.511038422848939078, 0.9923134781793048198 ) ) ;
#23842=DIRECTION ( 'NONE',  ( -3.002035892788116966E-16, 0.9996898646859343485, 0.02490330187381123786 ) ) ;
#23861=CARTESIAN_POINT ( 'NONE',  ( -61.34999999999997300, -2.583824419212624957, -0.5885162450438690129 ) ) ;
#23904=CARTESIAN_POINT ( 'NONE',  ( -61.38641854932647135, -2.625280434238165483, -0.6244966117725891941 ) ) ;
#23906=CIRCLE ( 'NONE', #31029, 2.685355339059328106 ) ;
#23916=CARTESIAN_POINT ( 'NONE',  ( -61.60260218697150236, -2.667562526553216795, 0.4270849601371985993 ) ) ;
#23922=CARTESIAN_POINT ( 'NONE',  ( -60.49999999999997868, 1.656632322739229403E-15, 1.870925083934595927E-15 ) ) ;
#23949=AXIS2_PLACEMENT_3D ( 'NONE', #27098, #19377, #10316 ) ;
#23967=CARTESIAN_POINT ( 'NONE',  ( -73.89999999999997726, -0.4598573377555323360, -0.01145551886194856595 ) ) ;
#23986=CARTESIAN_POINT ( 'NONE',  ( -60.59999999999997300, -2.458552378503722657, 0.9390651652154902163 ) ) ;
#24002=ORIENTED_EDGE ( 'NONE', *, *, #22387, .T. ) ;
#24007=TOROIDAL_SURFACE ( 'NONE', #10343, 2.649999999999999911, 0.05000000000000000278 ) ;
#24013=DIRECTION ( 'NONE',  ( 0.000000000000000000, -0.9996898646859343485, -0.02490330187381124133 ) ) ;
#24030=EDGE_LOOP ( 'NONE', ( #6918, #12890, #18289, #21213 ) ) ;
#24034=ORIENTED_EDGE ( 'NONE', *, *, #10347, .F. ) ;
#24040=DIRECTION ( 'NONE',  ( 0.000000000000000000, -0.9996898646859343485, -0.02490330187381143562 ) ) ;
#24056=AXIS2_PLACEMENT_3D ( 'NONE', #804, #15217, #1262 ) ;
#24058=CIRCLE ( 'NONE', #3330, 1.302039949377232331 ) ;
#24059=ADVANCED_FACE ( 'NONE', ( #15385 ), #22013, .T. ) ;
#24065=CARTESIAN_POINT ( 'NONE',  ( -62.06488485593400384, -2.667381432228959515, 0.2068147105598954205 ) ) ;
#24092=VERTEX_POINT ( 'NONE', #22230 ) ;
#24099=EDGE_CURVE ( 'NONE', #10647, #20935, #16948, .T. ) ;
#24128=AXIS2_PLACEMENT_3D ( 'NONE', #14250, #23444, #1732 ) ;
#24134=ORIENTED_EDGE ( 'NONE', *, *, #12347, .F. ) ;
#24160=AXIS2_PLACEMENT_3D ( 'NONE', #6603, #8794, #21018 ) ;
#24164=VERTEX_POINT ( 'NONE', #18254 ) ;
#24165=ORIENTED_EDGE ( 'NONE', *, *, #24706, .T. ) ;
#24175=CARTESIAN_POINT ( 'NONE',  ( -73.89999999999997726, -2.435524336289708093E-15, 4.607889071584891164E-15 ) ) ;
#24192=AXIS2_PLACEMENT_3D ( 'NONE', #16546, #14157, #9100 ) ;
#24202=DIRECTION ( 'NONE',  ( -1.000000000000000000, -3.053848253006669023E-16, 2.042510438544995415E-16 ) ) ;
#24203=VERTEX_POINT ( 'NONE', #13620 ) ;
#24230=CARTESIAN_POINT ( 'NONE',  ( -62.05074114918922845, -2.687605151338700704, 0.2580611626218518584 ) ) ;
#24234=CARTESIAN_POINT ( 'NONE',  ( -62.29999999999998295, 1.106939637198029038E-15, 2.238576962872695299E-15 ) ) ;
#24246=EDGE_CURVE ( 'NONE', #2409, #18413, #18400, .T. ) ;
#24250=VERTEX_POINT ( 'NONE', #3666 ) ;
#24268=CARTESIAN_POINT ( 'NONE',  ( -61.39999999999998437, -2.565822298769830478, -0.8405688140393350327 ) ) ;
#24283=ORIENTED_EDGE ( 'NONE', *, *, #12895, .F. ) ;
#24287=VERTEX_POINT ( 'NONE', #26148 ) ;
#24323=ORIENTED_EDGE ( 'NONE', *, *, #18414, .F. ) ;
#24338=EDGE_CURVE ( 'NONE', #2901, #28072, #6835, .T. ) ;
#24341=EDGE_CURVE ( 'NONE', #20831, #2488, #8824, .T. ) ;
#24363=DIRECTION ( 'NONE',  ( 0.000000000000000000, 0.9996898646859344595, 0.02490330187381124133 ) ) ;
#24424=CARTESIAN_POINT ( 'NONE',  ( -61.36293602036113271, -2.641650077464329005, 0.4741806564687899295 ) ) ;
#24441=CARTESIAN_POINT ( 'NONE',  ( -74.39999999999997726, -1.239615432210561474, -0.03088009432352123093 ) ) ;
#24450=DIRECTION ( 'NONE',  ( 0.000000000000000000, 0.9996898646859344595, 0.02490330187381105745 ) ) ;
#24457=CARTESIAN_POINT ( 'NONE',  ( -62.06710100716625789, -2.517118187348250213, 0.1993515260053453086 ) ) ;
#24466=EDGE_LOOP ( 'NONE', ( #16622, #4102, #31220, #19921 ) ) ;
#24509=AXIS2_PLACEMENT_3D ( 'NONE', #17965, #27614, #5942 ) ;
#24525=FACE_OUTER_BOUND ( 'NONE', #13055, .T. ) ;
#24530=CARTESIAN_POINT ( 'NONE',  ( -62.09999999999997300, -2.625757682666624238, -0.2804666419185134485 ) ) ;
#24538=DIRECTION ( 'NONE',  ( 0.000000000000000000, -0.9996898646859343485, -0.02490330187381124133 ) ) ;
#24557=CARTESIAN_POINT ( 'NONE',  ( -61.36066246949631875, -2.556345655048151144, -0.8088090313980157431 ) ) ;
#24563=VERTEX_POINT ( 'NONE', #6407 ) ;
#24573=ORIENTED_EDGE ( 'NONE', *, *, #12718, .T. ) ;
#24629=ORIENTED_EDGE ( 'NONE', *, *, #8812, .T. ) ;
#24649=AXIS2_PLACEMENT_3D ( 'NONE', #20254, #12932, #15791 ) ;
#24696=EDGE_LOOP ( 'NONE', ( #24922, #21411, #4132, #2030 ) ) ;
#24698=FACE_BOUND ( 'NONE', #16587, .T. ) ;
#24706=EDGE_CURVE ( 'NONE', #24164, #26416, #14488, .T. ) ;
#24720=CARTESIAN_POINT ( 'NONE',  ( -61.35074562499247008, -2.538044284739583656, -0.7956845220112261918 ) ) ;
#24727=CARTESIAN_POINT ( 'NONE',  ( -62.09999999999997300, 1.168016602258162478E-15, 2.197726754101795588E-15 ) ) ;
#24752=ORIENTED_EDGE ( 'NONE', *, *, #14924, .T. ) ;
#24774=CARTESIAN_POINT ( 'NONE',  ( -62.08896444478691024, -2.506042826205294283, -0.3088273841889361271 ) ) ;
#24777=CARTESIAN_POINT ( 'NONE',  ( -60.59999999999997300, -2.458552378503722657, 0.9390651652154902163 ) ) ;
#24823=DIRECTION ( 'NONE',  ( 0.000000000000000000, -0.9996898646859344595, -0.02490330187381124827 ) ) ;
#24824=DIRECTION ( 'NONE',  ( -1.000000000000000000, -3.053848253006669023E-16, 2.042510438544995415E-16 ) ) ;
#24825=CARTESIAN_POINT ( 'NONE',  ( -61.83175433005612120, -2.659179716902812629, -0.4747749904632609375 ) ) ;
#24826=CARTESIAN_POINT ( 'NONE',  ( -61.34999999999997300, -2.574153985709302539, -0.5872647410103332133 ) ) ;
#24832=CARTESIAN_POINT ( 'NONE',  ( -60.60352959746391122, -2.493729372996688731, 0.9514323440252360209 ) ) ;
#24864=EDGE_CURVE ( 'NONE', #24250, #22580, #4670, .T. ) ;
#24865=CARTESIAN_POINT ( 'NONE',  ( -62.04999999999998295, -2.687391533643777919, 0.2606275981160458555 ) ) ;
#24909=CARTESIAN_POINT ( 'NONE',  ( -61.09488783161975078, -2.409829088982875511, 0.7600985921382209520 ) ) ;
#24910=DIRECTION ( 'NONE',  ( 0.000000000000000000, 0.02490330187381123092, -0.9996898646859343485 ) ) ;
#24921=CARTESIAN_POINT ( 'NONE',  ( -61.39719200130745236, -2.604935742679383548, 0.7098721203061703067 ) ) ;
#24922=ORIENTED_EDGE ( 'NONE', *, *, #12289, .T. ) ;
#24952=( BOUNDED_CURVE ( )  B_SPLINE_CURVE ( 3, ( #762, #10885, #10427, #940 ),
 .UNSPECIFIED., .F., .F. ) 
 B_SPLINE_CURVE_WITH_KNOTS ( ( 4, 4 ),
 ( 1.362166255977964147, 1.466857099139255105 ),
 .UNSPECIFIED. ) 
 CURVE ( )  GEOMETRIC_REPRESENTATION_ITEM ( )  RATIONAL_B_SPLINE_CURVE ( ( 1.000000000000000000, 0.9990868608118155247, 0.9990868608118155247, 1.000000000000000000 ) ) 
 REPRESENTATION_ITEM ( '' )  );
#24978=EDGE_CURVE ( 'NONE', #24250, #2594, #3146, .T. ) ;
#24991=ORIENTED_EDGE ( 'NONE', *, *, #20299, .F. ) ;
#24994=FACE_OUTER_BOUND ( 'NONE', #18356, .T. ) ;
#25035=CARTESIAN_POINT ( 'NONE',  ( -62.14999999999998437, 1.152747360993128871E-15, 2.207939306294521009E-15 ) ) ;
#25038=DIRECTION ( 'NONE',  ( -1.000000000000000000, -3.053848253006669023E-16, 2.042510438544995415E-16 ) ) ;
#25041=( NAMED_UNIT ( * ) PLANE_ANGLE_UNIT ( ) SI_UNIT ( $, .RADIAN. ) );
#25078=CARTESIAN_POINT ( 'NONE',  ( -61.39798924013852854, -2.604827329856813645, 0.7104159706129550278 ) ) ;
#25085=CARTESIAN_POINT ( 'NONE',  ( -62.06710100716625789, -2.624587610216423172, -0.3274367013645053115 ) ) ;
#25086=EDGE_CURVE ( 'NONE', #6272, #3316, #22315, .T. ) ;
#25114=EDGE_CURVE ( 'NONE', #13929, #14583, #18026, .T. ) ;
#25154=CARTESIAN_POINT ( 'NONE',  ( -44.49999999999997868, 6.542789527549899840E-15, -1.397091617737396343E-15 ) ) ;
#25160=EDGE_LOOP ( 'NONE', ( #30897, #7546, #8674, #25726, #27939 ) ) ;
#25177=CARTESIAN_POINT ( 'NONE',  ( -73.89999999999997726, -2.435524336289708093E-15, 4.607889071584891164E-15 ) ) ;
#25178=AXIS2_PLACEMENT_3D ( 'NONE', #25553, #23679, #31090 ) ;
#25194=FACE_OUTER_BOUND ( 'NONE', #23456, .T. ) ;
#25214=EDGE_CURVE ( 'NONE', #1641, #30026, #14347, .T. ) ;
#25323=ORIENTED_EDGE ( 'NONE', *, *, #24246, .T. ) ;
#25325=DIRECTION ( 'NONE',  ( 3.002035892788116966E-16, -0.9996898646859343485, -0.02490330187381123786 ) ) ;
#25329=DIRECTION ( 'NONE',  ( 0.000000000000000000, -0.9996898646859343485, -0.02490330187381124133 ) ) ;
#25348=CARTESIAN_POINT ( 'NONE',  ( -62.09999999999997300, -2.720545749060828022, -0.4014110452728629763 ) ) ;
#25354=CARTESIAN_POINT ( 'NONE',  ( -44.49999999999997868, 0.7497673985144572839, 0.01867747640536023684 ) ) ;
#25358=DIRECTION ( 'NONE',  ( 0.000000000000000000, -0.9996898646859343485, -0.02490330187381124133 ) ) ;
#25384=FACE_OUTER_BOUND ( 'NONE', #5000, .T. ) ;
#25398=VERTEX_POINT ( 'NONE', #23967 ) ;
#25405=DIRECTION ( 'NONE',  ( 3.002035892788117459E-16, -0.9996898646859344595, -0.02490330187381124133 ) ) ;
#25422=EDGE_CURVE ( 'NONE', #30944, #9458, #28399, .T. ) ;
#25423=CARTESIAN_POINT ( 'NONE',  ( -73.90999999999998238, -2.438578184542714499E-15, 4.609931582023435380E-15 ) ) ;
#25427=ORIENTED_EDGE ( 'NONE', *, *, #8479, .T. ) ;
#25430=ORIENTED_EDGE ( 'NONE', *, *, #7926, .F. ) ;
#25435=ORIENTED_EDGE ( 'NONE', *, *, #27443, .T. ) ;
#25439=CARTESIAN_POINT ( 'NONE',  ( -74.39999999999997726, -2.588216748940040213E-15, 4.710014593512140639E-15 ) ) ;
#25448=AXIS2_PLACEMENT_3D ( 'NONE', #23922, #9681, #26768 ) ;
#25462=EDGE_LOOP ( 'NONE', ( #26891, #1675, #10172, #16813 ) ) ;
#25471=CARTESIAN_POINT ( 'NONE',  ( -44.49999999999997868, 6.542789527549899840E-15, -1.397091617737396343E-15 ) ) ;
#25476=EDGE_CURVE ( 'NONE', #24164, #18442, #26540, .T. ) ;
#25485=AXIS2_PLACEMENT_3D ( 'NONE', #9951, #26878, #14543 ) ;
#25491=DIRECTION ( 'NONE',  ( 3.002035892788117459E-16, -0.9996898646859343485, -0.02490330187381123786 ) ) ;
#25493=DIRECTION ( 'NONE',  ( 0.000000000000000000, -0.9996898646859343485, -0.02490330187381124133 ) ) ;
#25506=ORIENTED_EDGE ( 'NONE', *, *, #8474, .T. ) ;
#25544=DIRECTION ( 'NONE',  ( 0.000000000000000000, -0.9996898646859344595, -0.02490330187381124480 ) ) ;
#25553=CARTESIAN_POINT ( 'NONE',  ( -62.04999999999998295, -2.720545749060828022, -0.4014110452728629763 ) ) ;
#25554=DIRECTION ( 'NONE',  ( 0.000000000000000000, -0.9996898646859344595, -0.02490330187381124133 ) ) ;
#25567=FACE_OUTER_BOUND ( 'NONE', #13369, .T. ) ;
#25596=ORIENTED_EDGE ( 'NONE', *, *, #5530, .F. ) ;
#25626=ORIENTED_EDGE ( 'NONE', *, *, #19592, .T. ) ;
#25629=CIRCLE ( 'NONE', #24056, 0.04999999999999988481 ) ;
#25652=CYLINDRICAL_SURFACE ( 'NONE', #26131, 2.800000000000000266 ) ;
#25662=CARTESIAN_POINT ( 'NONE',  ( -62.06665691342191593, -2.643441408648605329, -0.3316822223133865100 ) ) ;
#25677=DIRECTION ( 'NONE',  ( -3.002035892788117459E-16, 0.9996898646859344595, 0.02490330187381124133 ) ) ;
#25678=ORIENTED_EDGE ( 'NONE', *, *, #16432, .T. ) ;
#25725=DIRECTION ( 'NONE',  ( 3.002035892788116966E-16, -0.9996898646859343485, -0.02490330187381123786 ) ) ;
#25726=ORIENTED_EDGE ( 'NONE', *, *, #14969, .F. ) ;
#25734=ADVANCED_FACE ( 'NONE', ( #25567 ), #26637, .T. ) ;
#25756=ORIENTED_EDGE ( 'NONE', *, *, #5611, .T. ) ;
#25757=CARTESIAN_POINT ( 'NONE',  ( -63.82928932188132620, -2.649178141417726451, -0.06599374996559692619 ) ) ;
#25789=ORIENTED_EDGE ( 'NONE', *, *, #13713, .T. ) ;
#25797=CARTESIAN_POINT ( 'NONE',  ( -61.39999999999998437, -2.624491116890564690, -0.6340712715164679159 ) ) ;
#25798=( BOUNDED_CURVE ( )  B_SPLINE_CURVE ( 3, ( #24865, #27253, #27724, #20152 ),
 .UNSPECIFIED., .F., .T. ) 
 B_SPLINE_CURVE_WITH_KNOTS ( ( 4, 4 ),
 ( 4.833974135028384467, 4.924538311792051815 ),
 .UNSPECIFIED. ) 
 CURVE ( )  GEOMETRIC_REPRESENTATION_ITEM ( )  RATIONAL_B_SPLINE_CURVE ( ( 1.000000000000000000, 0.9993166276053078168, 0.9993166276053078168, 1.000000000000000000 ) ) 
 REPRESENTATION_ITEM ( '' )  );
#25852=CARTESIAN_POINT ( 'NONE',  ( -61.34999999999997300, -2.635021238245644160, -0.5887810068220489246 ) ) ;
#25857=DIRECTION ( 'NONE',  ( 1.000000000000000000, 3.053848253006669023E-16, -2.042510438544995169E-16 ) ) ;
#25859=ORIENTED_EDGE ( 'NONE', *, *, #26532, .T. ) ;
#25863=ORIENTED_EDGE ( 'NONE', *, *, #25086, .T. ) ;
#25896=ORIENTED_EDGE ( 'NONE', *, *, #22127, .F. ) ;
#25903=CARTESIAN_POINT ( 'NONE',  ( -61.34999999999997300, -2.456456838093036055, -0.5843327841101846332 ) ) ;
#25939=VERTEX_POINT ( 'NONE', #1307 ) ;
#25946=DIRECTION ( 'NONE',  ( 0.000000000000000000, -0.9996898646859343485, -0.02490330187381124133 ) ) ;
#25953=CARTESIAN_POINT ( 'NONE',  ( -62.05955358283408430, -2.690595597012027884, 0.2275897585651485699 ) ) ;
#25961=LINE ( 'NONE', #13603, #21123 ) ;
#25987=CARTESIAN_POINT ( 'NONE',  ( 0.000000000000000000, 0.000000000000000000, 0.000000000000000000 ) ) ;
#25995=CARTESIAN_POINT ( 'NONE',  ( -60.59999999999997300, 1.626093840209163176E-15, 1.891350188320046374E-15 ) ) ;
#26027=PLANE ( 'NONE',  #11126 ) ;
#26032=CARTESIAN_POINT ( 'NONE',  ( -62.09999999999997300, -2.733115994082214950, 0.2227785043249702612 ) ) ;
#26054=MANIFOLD_SOLID_BREP ( 'Stock-MAS-683-1', #30700 ) ;
#26078=VECTOR ( 'NONE', #766, 1000.000000000000000 ) ;
#26097=DIRECTION ( 'NONE',  ( 2.117927888850091331E-16, -0.02490330187381135929, 0.9996898646859343485 ) ) ;
#26126=FACE_OUTER_BOUND ( 'NONE', #8454, .T. ) ;
#26131=AXIS2_PLACEMENT_3D ( 'NONE', #28668, #15989, #30880 ) ;
#26148=CARTESIAN_POINT ( 'NONE',  ( -60.49999999999997868, 2.624185894800579621, 0.06537116741875470538 ) ) ;
#26163=AXIS2_PLACEMENT_3D ( 'NONE', #5514, #15004, #15169 ) ;
#26173=CARTESIAN_POINT ( 'NONE',  ( -74.38999999999998636, -2.585162900687033808E-15, 4.707972083073595634E-15 ) ) ;
#26194=ORIENTED_EDGE ( 'NONE', *, *, #9789, .F. ) ;
#26263=ORIENTED_EDGE ( 'NONE', *, *, #6137, .F. ) ;
#26280=ORIENTED_EDGE ( 'NONE', *, *, #5877, .F. ) ;
#26291=CARTESIAN_POINT ( 'NONE',  ( -60.59999999999997300, -2.342723651847746336, 0.9419505778294103848 ) ) ;
#26292=CARTESIAN_POINT ( 'NONE',  ( -62.05955090584385658, -2.675925004799827978, -0.3612845363725897263 ) ) ;
#26293=AXIS2_PLACEMENT_3D ( 'NONE', #19885, #29516, #7830 ) ;
#26296=ORIENTED_EDGE ( 'NONE', *, *, #8479, .F. ) ;
#26311=CARTESIAN_POINT ( 'NONE',  ( -73.90999999999998238, 1.249612330857415632, 0.03112912734226871286 ) ) ;
#26319=ORIENTED_EDGE ( 'NONE', *, *, #18783, .T. ) ;
#26326=PRESENTATION_STYLE_ASSIGNMENT (( #18895 ) ) ;
#26329=CARTESIAN_POINT ( 'NONE',  ( -62.14999999999998437, 2.749147127886321318, 0.06848408015298346196 ) ) ;
#26333=DIRECTION ( 'NONE',  ( -1.000000000000000000, -3.053848253006669023E-16, 2.042510438544995415E-16 ) ) ;
#26381=ORIENTED_EDGE ( 'NONE', *, *, #8115, .T. ) ;
#26385=EDGE_CURVE ( 'NONE', #13383, #18442, #25798, .T. ) ;
#26386=CARTESIAN_POINT ( 'NONE',  ( -74.38999999999998636, 1.249612330857415410, 0.03112912734226870939 ) ) ;
#26390=ORIENTED_EDGE ( 'NONE', *, *, #2490, .T. ) ;
#26393=DIRECTION ( 'NONE',  ( -3.002035892788117459E-16, 0.9996898646859344595, 0.02490330187381124133 ) ) ;
#26400=ADVANCED_FACE ( 'NONE', ( #12675 ), #12995, .T. ) ;
#26405=DIRECTION ( 'NONE',  ( -1.000000000000000000, -3.053848253006669023E-16, 2.042510438544995415E-16 ) ) ;
#26416=VERTEX_POINT ( 'NONE', #5878 ) ;
#26442=EDGE_CURVE ( 'NONE', #13516, #23278, #5569, .T. ) ;
#26453=ORIENTED_EDGE ( 'NONE', *, *, #16432, .F. ) ;
#26460=DIRECTION ( 'NONE',  ( 0.000000000000000000, 0.9996898646859344595, 0.02490330187381124133 ) ) ;
#26473=CARTESIAN_POINT ( 'NONE',  ( -61.13542439536082895, -2.534004151299444896, -0.9379212110198712482 ) ) ;
#26475=CARTESIAN_POINT ( 'NONE',  ( -61.34999999999997300, -2.528827883897363904, -0.7921676171260561006 ) ) ;
#26484=CARTESIAN_POINT ( 'NONE',  ( -67.34999999999998010, -4.352537305703398686E-16, 3.270044734337918230E-15 ) ) ;
#26509=DIRECTION ( 'NONE',  ( -1.000000000000000000, -3.053848253006669023E-16, 2.042510438544995415E-16 ) ) ;
#26511=AXIS2_PLACEMENT_3D ( 'NONE', #22790, #22930, #15322 ) ;
#26515=DIRECTION ( 'NONE',  ( 0.000000000000000000, 0.9996898646859344595, 0.02490330187381124480 ) ) ;
#26532=EDGE_CURVE ( 'NONE', #26416, #1831, #25961, .T. ) ;
#26540=B_SPLINE_CURVE_WITH_KNOTS ( 'NONE', 3,
 ( #13968, #21301, #27421, #22520, #514, #27103, #14909, #10171, #24424, #2891, #2735, #10321, #12541, #29470, #29796, #3196, #661, #7784, #19539, #8111, #19840, #5585 ),
 .UNSPECIFIED., .F., .F.,
 ( 4, 3, 3, 3, 3, 3, 3, 4 ),
 ( 0.000000000000000000, 1.393664602030251122E-05, 2.794505907987546679E-05, 4.337356477558444669E-05, 6.134619026776088897E-05, 8.251722506675484789E-05, 8.560979848730156062E-05, 8.708485877085708770E-05 ),
 .UNSPECIFIED. ) ;
#26542=AXIS2_PLACEMENT_3D ( 'NONE', #9217, #18877, #26460 ) ;
#26563=CARTESIAN_POINT ( 'NONE',  ( -61.57738852934189566, -2.654103483775546390, -0.5064680332891128289 ) ) ;
#26569=LINE ( 'NONE', #12173, #4431 ) ;
#26577=AXIS2_PLACEMENT_3D ( 'NONE', #9571, #26333, #7638 ) ;
#26591=CARTESIAN_POINT ( 'NONE',  ( -62.05495586881989567, -2.687269152040965725, 0.2433159615545962828 ) ) ;
#26611=AXIS2_PLACEMENT_3D ( 'NONE', #24234, #10125, #12642 ) ;
#26621=VERTEX_POINT ( 'NONE', #3266 ) ;
#26623=CIRCLE ( 'NONE', #3440, 0.04999999999999988481 ) ;
#26631=CIRCLE ( 'NONE', #30167, 0.05000000000000001665 ) ;
#26637=( BOUNDED_SURFACE ( )  B_SPLINE_SURFACE ( 3, 2, ( 
 ( #5969, #22595, #13072 ),
 ( #20699, #30470, #20383 ),
 ( #11022, #8631, #8774 ),
 ( #22758, #18466, #23219 ) ),
 .UNSPECIFIED., .F., .F., .F. ) 
 B_SPLINE_SURFACE_WITH_KNOTS ( ( 4, 4 ),
 ( 3, 3 ),
 ( 1.163945177512966334, 1.279805501628815900 ),
 ( 0.000000000000000000, 1.000000000000000000 ),
 .UNSPECIFIED. ) 
 GEOMETRIC_REPRESENTATION_ITEM ( )  RATIONAL_B_SPLINE_SURFACE ( (
 ( 1.000000000000000000, 0.5604218610591209515, 1.000000000000000000),
 ( 1.000000000000000000, 0.5752896509278202508, 1.000000000000000000),
 ( 1.000000000000000000, 0.5899361674293628344, 1.000000000000000000),
 ( 1.000000000000000000, 0.6043181045777068494, 1.000000000000000000) ) ) 
 REPRESENTATION_ITEM ( '' )  SURFACE ( )  );
#26658=EDGE_CURVE ( 'NONE', #23537, #28771, #2907, .T. ) ;
#26660=EDGE_LOOP ( 'NONE', ( #15813, #11212, #2993, #18776, #27200, #27813 ) ) ;
#26686=TOROIDAL_SURFACE ( 'NONE', #16042, 2.649999999999999911, 0.05000000000000000278 ) ;
#26691=ADVANCED_FACE ( 'NONE', ( #12909 ), #23785, .T. ) ;
#26693=FACE_OUTER_BOUND ( 'NONE', #24030, .T. ) ;
#26694=CIRCLE ( 'NONE', #4935, 1.250000000000000222 ) ;
#26700=ORIENTED_EDGE ( 'NONE', *, *, #7399, .T. ) ;
#26721=DIRECTION ( 'NONE',  ( -0.9396926207859095381, -0.008517430876163519654, 0.3419140708010985352 ) ) ;
#26741=CARTESIAN_POINT ( 'NONE',  ( -61.36283645075994286, -2.621142715471549423, -0.6477737761984685427 ) ) ;
#26749=DIRECTION ( 'NONE',  ( 1.000000000000000000, 3.053848253006669023E-16, -2.042510438544995415E-16 ) ) ;
#26768=DIRECTION ( 'NONE',  ( 0.000000000000000000, -0.9996898646859344595, -0.02490330187381124133 ) ) ;
#26774=EDGE_LOOP ( 'NONE', ( #24991, #16790, #2441, #18290 ) ) ;
#26797=CARTESIAN_POINT ( 'NONE',  ( -61.34999999999997300, -2.515554072771550853, -0.7899129066418597578 ) ) ;
#26845=ORIENTED_EDGE ( 'NONE', *, *, #7519, .T. ) ;
#26862=CARTESIAN_POINT ( 'NONE',  ( -62.29999999999998295, 1.106939637198029038E-15, 2.238576962872695299E-15 ) ) ;
#26878=DIRECTION ( 'NONE',  ( 1.000000000000000000, 3.053848253006669023E-16, -2.042510438544995415E-16 ) ) ;
#26891=ORIENTED_EDGE ( 'NONE', *, *, #18193, .T. ) ;
#26986=DIRECTION ( 'NONE',  ( 3.002035892788116966E-16, -0.9996898646859343485, -0.02490330187381123786 ) ) ;
#27010=EDGE_CURVE ( 'NONE', #29446, #3131, #14546, .T. ) ;
#27015=VERTEX_POINT ( 'NONE', #12722 ) ;
#27019=CONICAL_SURFACE ( 'NONE', #13357, 1.600000000000000533, 0.7853981633974497223 ) ;
#27028=CARTESIAN_POINT ( 'NONE',  ( -60.59999999999997300, -2.426837276046140079, -1.064406330116907329 ) ) ;
#27095=TOROIDAL_SURFACE ( 'NONE', #7975, 1.239999999999999991, 0.01000000000000000021 ) ;
#27097=VECTOR ( 'NONE', #27362, 1000.000000000000000 ) ;
#27098=CARTESIAN_POINT ( 'NONE',  ( -62.09999999999997300, -2.693793069130350659, 0.1829724042179160792 ) ) ;
#27103=CARTESIAN_POINT ( 'NONE',  ( -61.35505088056748235, -2.631273283024623488, 0.4666624523549950943 ) ) ;
#27108=B_SPLINE_CURVE_WITH_KNOTS ( 'NONE', 3,
 ( #15166, #19926, #29729, #27028 ),
 .UNSPECIFIED., .F., .F.,
 ( 4, 4 ),
 ( 0.000000000000000000, 1.854844919671800558E-05 ),
 .UNSPECIFIED. ) ;
#27130=CARTESIAN_POINT ( 'NONE',  ( -61.34999999999997300, -2.524557112582767715, -0.7907883100310012514 ) ) ;
#27146=CIRCLE ( 'NONE', #31124, 2.525000000000001243 ) ;
#27167=ADVANCED_FACE ( 'NONE', ( #26693 ), #29667, .F. ) ;
#27180=ADVANCED_FACE ( 'NONE', ( #4990 ), #14646, .T. ) ;
#27188=CARTESIAN_POINT ( 'NONE',  ( -60.64999999999998437, -2.511038422848939078, 0.9923134781793048198 ) ) ;
#27200=ORIENTED_EDGE ( 'NONE', *, *, #5571, .F. ) ;
#27211=CARTESIAN_POINT ( 'NONE',  ( -62.09999999999997300, -2.737380368259866525, 0.2631615932906978261 ) ) ;
#27215=LINE ( 'NONE', #27512, #23064 ) ;
#27223=ORIENTED_EDGE ( 'NONE', *, *, #22127, .T. ) ;
#27225=CARTESIAN_POINT ( 'NONE',  ( -62.34999999999997300, -2.749147127886318653, -0.06848408015297867413 ) ) ;
#27229=ORIENTED_EDGE ( 'NONE', *, *, #18602, .T. ) ;
#27251=DIRECTION ( 'NONE',  ( 0.000000000000000000, 0.9996898646859344595, 0.02490330187381124133 ) ) ;
#27253=CARTESIAN_POINT ( 'NONE',  ( -61.83175433005612120, -2.679521002368077998, 0.3417824691599675724 ) ) ;
#27255=CARTESIAN_POINT ( 'NONE',  ( -62.08167832910348238, -2.517763198270825065, 0.1910326606448936038 ) ) ;
#27259=ORIENTED_EDGE ( 'NONE', *, *, #5571, .T. ) ;
#27262=CIRCLE ( 'NONE', #1982, 2.750000000000000444 ) ;
#27270=EDGE_CURVE ( 'NONE', #22178, #4534, #17019, .T. ) ;
#27271=ORIENTED_EDGE ( 'NONE', *, *, #427, .F. ) ;
#27276=CARTESIAN_POINT ( 'NONE',  ( -74.39999999999997726, -2.588216748940040213E-15, 4.710014593512140639E-15 ) ) ;
#27278=DIRECTION ( 'NONE',  ( 0.000000000000000000, -0.9996898646859344595, -0.02490330187381124480 ) ) ;
#27309=CARTESIAN_POINT ( 'NONE',  ( -62.07031753968892218, -2.504221380502570593, -0.3232671695957713975 ) ) ;
#27312=CARTESIAN_POINT ( 'NONE',  ( -61.37941297909985394, -2.603941716553896946, 0.6968202940837837644 ) ) ;
#27328=CARTESIAN_POINT ( 'NONE',  ( -67.91948434493399134, 1.598692187574554335, 0.03982506530961366781 ) ) ;
#27333=CARTESIAN_POINT ( 'NONE',  ( -61.34138854390450035, -2.661151313430901943, 0.4599831919335348185 ) ) ;
#27353=EDGE_LOOP ( 'NONE', ( #23007, #1179, #11838, #6880, #9942 ) ) ;
#27362=DIRECTION ( 'NONE',  ( 1.000000000000000000, 3.053848253006669023E-16, -2.042510438544995415E-16 ) ) ;
#27404=CIRCLE ( 'NONE', #6173, 2.525000000000001243 ) ;
#27421=CARTESIAN_POINT ( 'NONE',  ( -61.35067034588222867, -2.619031987328097610, 0.4612939446252454778 ) ) ;
#27423=EDGE_LOOP ( 'NONE', ( #12500, #814, #2079, #21899 ) ) ;
#27441=TOROIDAL_SURFACE ( 'NONE', #11785, 1.649144805949033898, 0.05000000000000000278 ) ;
#27443=EDGE_CURVE ( 'NONE', #11715, #25939, #19832, .T. ) ;
#27459=CARTESIAN_POINT ( 'NONE',  ( -61.35508841351263953, -2.585893814015340020, 0.6744937573145690646 ) ) ;
#27464=DIRECTION ( 'NONE',  ( -1.000000000000000000, -3.053848253006669023E-16, 2.042510438544995415E-16 ) ) ;
#27468=CARTESIAN_POINT ( 'NONE',  ( -61.34999999999997300, -2.556251174960431971, 0.6635690258132532771 ) ) ;
#27512=CARTESIAN_POINT ( 'NONE',  ( -73.89999999999997726, -0.4598573377555323360, -0.01145551886194856595 ) ) ;
#27550=DIRECTION ( 'NONE',  ( 1.000000000000000000, 3.053848253006669023E-16, -2.042510438544995415E-16 ) ) ;
#27554=LINE ( 'NONE', #22686, #16512 ) ;
#27568=AXIS2_PLACEMENT_3D ( 'NONE', #19255, #1979, #11951 ) ;
#27576=ORIENTED_EDGE ( 'NONE', *, *, #22498, .T. ) ;
#27592=CARTESIAN_POINT ( 'NONE',  ( -62.04999999999998295, 1.183285843523195887E-15, 2.187514201909070562E-15 ) ) ;
#27599=DIRECTION ( 'NONE',  ( -3.002035892788117459E-16, 0.9996898646859344595, 0.02490330187381124133 ) ) ;
#27609=VECTOR ( 'NONE', #5104, 1000.000000000000227 ) ;
#27613=ORIENTED_EDGE ( 'NONE', *, *, #15805, .T. ) ;
#27614=DIRECTION ( 'NONE',  ( 1.000000000000000000, 3.053848253006669023E-16, -2.042510438544995415E-16 ) ) ;
#27645=AXIS2_PLACEMENT_3D ( 'NONE', #26329, #4628, #2250 ) ;
#27666=ADVANCED_FACE ( 'NONE', ( #18710 ), #22103, .T. ) ;
#27672=EDGE_CURVE ( 'NONE', #10954, #23278, #26631, .T. ) ;
#27686=AXIS2_PLACEMENT_3D ( 'NONE', #21955, #17499, #26986 ) ;
#27687=CARTESIAN_POINT ( 'NONE',  ( -60.61395381780661751, -2.505988366243331100, 0.9638607592909542721 ) ) ;
#27701=ORIENTED_EDGE ( 'NONE', *, *, #10888, .F. ) ;
#27702=FACE_OUTER_BOUND ( 'NONE', #19348, .T. ) ;
#27704=FACE_BOUND ( 'NONE', #13979, .T. ) ;
#27707=CARTESIAN_POINT ( 'NONE',  ( -61.34999999999997300, -2.661068980108069137, 0.4568499568858441773 ) ) ;
#27713=CIRCLE ( 'NONE', #24192, 0.04999999999999988481 ) ;
#27715=TOROIDAL_SURFACE ( 'NONE', #12462, 2.649999999999999911, 0.05000000000000000278 ) ;
#27724=CARTESIAN_POINT ( 'NONE',  ( -61.61493949811855231, -2.667984932540325094, 0.4224978793964678236 ) ) ;
#27754=STYLED_ITEM ( 'NONE', ( #1290 ), #10428 ) ;
#27808=EDGE_CURVE ( 'NONE', #1827, #28152, #12962, .T. ) ;
#27813=ORIENTED_EDGE ( 'NONE', *, *, #16946, .F. ) ;
#27820=DIRECTION ( 'NONE',  ( 1.000000000000000000, 3.053848253006669023E-16, -2.042510438544995415E-16 ) ) ;
#27825=EDGE_CURVE ( 'NONE', #23465, #8800, #29161, .T. ) ;
#27826=EDGE_LOOP ( 'NONE', ( #668, #23672 ) ) ;
#27835=CARTESIAN_POINT ( 'NONE',  ( -62.29999999999998295, 1.106939637198029038E-15, 2.238576962872695299E-15 ) ) ;
#27836=AXIS2_PLACEMENT_3D ( 'NONE', #16549, #9591, #19088 ) ;
#27860=FACE_OUTER_BOUND ( 'NONE', #8933, .T. ) ;
#27879=CARTESIAN_POINT ( 'NONE',  ( -62.34999999999997300, 1.091670395932995432E-15, 2.248789515065420326E-15 ) ) ;
#27889=CARTESIAN_POINT ( 'NONE',  ( -60.60352959746391122, -2.443263361361769803, -1.074417906603847728 ) ) ;
#27909=CARTESIAN_POINT ( 'NONE',  ( -62.06710100716625789, -2.517118187348250213, 0.1993515260053453086 ) ) ;
#27915=CARTESIAN_POINT ( 'NONE',  ( -62.04999999999998295, -2.687391533643777919, 0.2606275981160458555 ) ) ;
#27920=ORIENTED_EDGE ( 'NONE', *, *, #20299, .T. ) ;
#27926=FACE_OUTER_BOUND ( 'NONE', #29142, .T. ) ;
#27938=DIRECTION ( 'NONE',  ( -1.000000000000000000, -3.053848253006669023E-16, 2.042510438544995169E-16 ) ) ;
#27939=ORIENTED_EDGE ( 'NONE', *, *, #17070, .F. ) ;
#27968=DIRECTION ( 'NONE',  ( -1.000000000000000000, -3.053848253006669023E-16, 2.042510438544995415E-16 ) ) ;
#28020=DIRECTION ( 'NONE',  ( 3.002035892788117459E-16, -0.9996898646859344595, -0.02490330187381124133 ) ) ;
#28021=DIRECTION ( 'NONE',  ( 0.9994629430332293563, -0.03275911391080271046, -0.0008160631928541098616 ) ) ;
#28025=CARTESIAN_POINT ( 'NONE',  ( -62.09999999999997300, -2.700242798440558367, -0.3182811450455869662 ) ) ;
#28027=CARTESIAN_POINT ( 'NONE',  ( -62.04999999999998295, -2.671081280896084653, -0.3941126626315437642 ) ) ;
#28037=CARTESIAN_POINT ( 'NONE',  ( -60.59999999999997300, -2.532112727260102947, 0.9372327013327054201 ) ) ;
#28043=SHAPE_REPRESENTATION_RELATIONSHIP ( 'NONE' , 'NONE' ,  #29923, #10428 ) ;
#28060=CARTESIAN_POINT ( 'NONE',  ( -62.09999999999997300, 0.005353951483536216298, -0.2149229472152333620 ) ) ;
#28063=DIRECTION ( 'NONE',  ( 0.000000000000000000, 0.9996898646859343485, 0.02490330187381123439 ) ) ;
#28066=CARTESIAN_POINT ( 'NONE',  ( -61.34999999999997300, -2.581364933566181019, -0.7915523228156536861 ) ) ;
#28072=VERTEX_POINT ( 'NONE', #2027 ) ;
#28092=ORIENTED_EDGE ( 'NONE', *, *, #14666, .F. ) ;
#28109=CARTESIAN_POINT ( 'NONE',  ( -74.38999999999998636, -1.249612330857420739, -0.03112912734225924821 ) ) ;
#28116=EDGE_LOOP ( 'NONE', ( #21469, #26845, #31272, #2635 ) ) ;
#28122=ORIENTED_EDGE ( 'NONE', *, *, #25214, .T. ) ;
#28126=DIRECTION ( 'NONE',  ( -2.117927888850090838E-16, 0.02490330187381123786, -0.9996898646859343485 ) ) ;
#28152=VERTEX_POINT ( 'NONE', #16130 ) ;
#28155=ORIENTED_EDGE ( 'NONE', *, *, #27808, .F. ) ;
#28164=AXIS2_PLACEMENT_3D ( 'NONE', #21554, #29533, #8025 ) ;
#28167=AXIS2_PLACEMENT_3D ( 'NONE', #3683, #16037, #16198 ) ;
#28177=CARTESIAN_POINT ( 'NONE',  ( -62.09999999999998010, -2.637337459618612101, 0.1843787714682001699 ) ) ;
#28178=CIRCLE ( 'NONE', #1899, 0.05000000000000009298 ) ;
#28183=VECTOR ( 'NONE', #13296, 1000.000000000000000 ) ;
#28198=ORIENTED_EDGE ( 'NONE', *, *, #26442, .T. ) ;
#28211=( BOUNDED_CURVE ( )  B_SPLINE_CURVE ( 3, ( #19868, #24909, #8138, #15585 ),
 .UNSPECIFIED., .F., .T. ) 
 B_SPLINE_CURVE_WITH_KNOTS ( ( 4, 4 ),
 ( 5.004453192798488104, 5.119588733684844684 ),
 .UNSPECIFIED. ) 
 CURVE ( )  GEOMETRIC_REPRESENTATION_ITEM ( )  RATIONAL_B_SPLINE_CURVE ( ( 1.000000000000000000, 0.9988956223160183612, 0.9988956223160183612, 1.000000000000000000 ) ) 
 REPRESENTATION_ITEM ( '' )  );
#28228=DIRECTION ( 'NONE',  ( 1.000000000000000000, 3.053848253006669023E-16, -2.042510438544995415E-16 ) ) ;
#28250=EDGE_LOOP ( 'NONE', ( #9896, #27259, #4135, #30423, #18634, #19529 ) ) ;
#28258=DIRECTION ( 'NONE',  ( 2.117927888850091331E-16, -0.02490330187381135929, 0.9996898646859343485 ) ) ;
#28262=ORIENTED_EDGE ( 'NONE', *, *, #6548, .F. ) ;
#28264=CARTESIAN_POINT ( 'NONE',  ( -62.09999999999997300, -2.704716430269783700, 0.1751800441595645352 ) ) ;
#28288=DIRECTION ( 'NONE',  ( 0.000000000000000000, -0.9996898646859343485, -0.02490330187381143562 ) ) ;
#28295=AXIS2_PLACEMENT_3D ( 'NONE', #784, #20132, #5696 ) ;
#28309=CIRCLE ( 'NONE', #17689, 1.250000000000000222 ) ;
#28321=AXIS2_PLACEMENT_3D ( 'NONE', #8790, #30819, #28288 ) ;
#28328=ORIENTED_EDGE ( 'NONE', *, *, #12507, .T. ) ;
#28338=CARTESIAN_POINT ( 'NONE',  ( -61.35349513024766566, -2.601746391104207135, -0.5952655458314711767 ) ) ;
#28344=DIRECTION ( 'NONE',  ( -2.117927888850090838E-16, 0.02490330187381123786, -0.9996898646859343485 ) ) ;
#28349=EDGE_CURVE ( 'NONE', #23465, #29446, #20164, .T. ) ;
#28352=CARTESIAN_POINT ( 'NONE',  ( -62.09999999999998010, -2.624885808681706845, -0.3154661608747524326 ) ) ;
#28357=( BOUNDED_CURVE ( )  B_SPLINE_CURVE ( 3, ( #31065, #2097, #9239, #14130 ),
 .UNSPECIFIED., .F., .T. ) 
 B_SPLINE_CURVE_WITH_KNOTS ( ( 4, 4 ),
 ( 1.163596573494744213, 1.278732114381100571 ),
 .UNSPECIFIED. ) 
 CURVE ( )  GEOMETRIC_REPRESENTATION_ITEM ( )  RATIONAL_B_SPLINE_CURVE ( ( 1.000000000000000000, 0.9988956223160183612, 0.9988956223160183612, 1.000000000000000000 ) ) 
 REPRESENTATION_ITEM ( '' )  );
#28359=DIRECTION ( 'NONE',  ( 0.7071067811865466846, -0.7068874824028871240, -0.01760929362890767402 ) ) ;
#28374=ORIENTED_EDGE ( 'NONE', *, *, #12289, .F. ) ;
#28399=LINE ( 'NONE', #11772, #12446 ) ;
#28400=AXIS2_PLACEMENT_3D ( 'NONE', #18120, #15254, #2916 ) ;
#28413=CARTESIAN_POINT ( 'NONE',  ( -62.39999999999998437, 2.749147127886321318, 0.06848408015298351748 ) ) ;
#28438=ORIENTED_EDGE ( 'NONE', *, *, #10014, .T. ) ;
#28449=ORIENTED_EDGE ( 'NONE', *, *, #23497, .T. ) ;
#28478=CARTESIAN_POINT ( 'NONE',  ( -64.32138495697122949, 2.298612619042725846, 0.05726080253995516345 ) ) ;
#28512=DIRECTION ( 'NONE',  ( -3.002035892788117459E-16, 0.9996898646859344595, 0.02490330187381124133 ) ) ;
#28528=AXIS2_PLACEMENT_3D ( 'NONE', #15346, #15677, #13267 ) ;
#28567=FACE_OUTER_BOUND ( 'NONE', #10033, .T. ) ;
#28600=ORIENTED_EDGE ( 'NONE', *, *, #27270, .F. ) ;
#28605=ORIENTED_EDGE ( 'NONE', *, *, #18193, .F. ) ;
#28616=PLANE ( 'NONE',  #4624 ) ;
#28651=CARTESIAN_POINT ( 'NONE',  ( -74.38999999999998636, -2.585162900687033808E-15, 4.707972083073595634E-15 ) ) ;
#28668=CARTESIAN_POINT ( 'NONE',  ( -62.34999999999997300, 1.091670395932995432E-15, 2.248789515065420326E-15 ) ) ;
#28676=DIRECTION ( 'NONE',  ( 1.000000000000000000, 3.053848253006669023E-16, -2.042510438544995415E-16 ) ) ;
#28678=VERTEX_POINT ( 'NONE', #24530 ) ;
#28689=DIRECTION ( 'NONE',  ( -1.000000000000000000, -3.053848253006669023E-16, 2.042510438544995415E-16 ) ) ;
#28716=EDGE_CURVE ( 'NONE', #11715, #20935, #1903, .T. ) ;
#28721=VERTEX_POINT ( 'NONE', #6940 ) ;
#28771=VERTEX_POINT ( 'NONE', #30841 ) ;
#28812=CARTESIAN_POINT ( 'NONE',  ( -62.04999999999998295, -2.737158043526071172, 0.2654540351181890467 ) ) ;
#28846=ORIENTED_EDGE ( 'NONE', *, *, #13839, .T. ) ;
#28860=CARTESIAN_POINT ( 'NONE',  ( -60.61250724947091584, -2.452226114303401427, -1.129861533254596928 ) ) ;
#28881=ORIENTED_EDGE ( 'NONE', *, *, #22364, .T. ) ;
#28896=CARTESIAN_POINT ( 'NONE',  ( -60.89492752328840908, -2.547300119769525750, 0.9005536500125419508 ) ) ;
#28897=CARTESIAN_POINT ( 'NONE',  ( -62.04999999999998295, -2.625757682666624238, -0.2804666419185135040 ) ) ;
#28941=ORIENTED_EDGE ( 'NONE', *, *, #7519, .F. ) ;
#28958=DIRECTION ( 'NONE',  ( -1.000000000000000000, -3.053848253006669023E-16, 2.042510438544995169E-16 ) ) ;
#28969=CARTESIAN_POINT ( 'NONE',  ( -62.06682860016772452, -2.653360696315357092, 0.1987474702245471680 ) ) ;
#28984=ORIENTED_EDGE ( 'NONE', *, *, #29379, .T. ) ;
#28986=B_SPLINE_CURVE_WITH_KNOTS ( 'NONE', 3,
 ( #28027, #30889, #16477, #16001, #4446, #14096, #13611, #1271, #11096, #20776, #30402, #25662, #3971, #23301, #11243, #30553 ),
 .UNSPECIFIED., .F., .F.,
 ( 4, 3, 3, 3, 3, 4 ),
 ( 0.000000000000000000, 2.177138635050367827E-05, 4.299041441261427111E-05, 6.255873377259018090E-05, 8.005453962339759144E-05, 9.359446731969179928E-05 ),
 .UNSPECIFIED. ) ;
#29015=CARTESIAN_POINT ( 'NONE',  ( -61.34999999999997300, -2.581364933566181019, -0.7915523228156536861 ) ) ;
#29038=TOROIDAL_SURFACE ( 'NONE', #15368, 2.100674278852607824, 0.05000000000000000278 ) ;
#29072=ORIENTED_EDGE ( 'NONE', *, *, #13067, .T. ) ;
#29088=EDGE_LOOP ( 'NONE', ( #8215, #13017, #25863, #3976 ) ) ;
#29111=DIRECTION ( 'NONE',  ( -1.000000000000000000, -3.053848253006669023E-16, 2.042510438544995415E-16 ) ) ;
#29136=LINE ( 'NONE', #14576, #23687 ) ;
#29142=EDGE_LOOP ( 'NONE', ( #2099, #10326, #18919, #8783 ) ) ;
#29155=CIRCLE ( 'NONE', #4379, 2.750000000000000444 ) ;
#29161=CIRCLE ( 'NONE', #24128, 0.01000000000000001929 ) ;
#29201=CARTESIAN_POINT ( 'NONE',  ( -62.29999999999998295, -2.799131621120614977, -0.06972924524666890278 ) ) ;
#29216=TOROIDAL_SURFACE ( 'NONE', #23170, 1.260000000000000009, 0.01000000000000000021 ) ;
#29228=ORIENTED_EDGE ( 'NONE', *, *, #2889, .T. ) ;
#29229=FACE_OUTER_BOUND ( 'NONE', #29344, .T. ) ;
#29248=AXIS2_PLACEMENT_3D ( 'NONE', #23777, #16479, #23449 ) ;
#29258=ORIENTED_EDGE ( 'NONE', *, *, #2208, .F. ) ;
#29263=CARTESIAN_POINT ( 'NONE',  ( -62.06968758346935999, -2.680528337278641704, -0.3278885135174935961 ) ) ;
#29272=CARTESIAN_POINT ( 'NONE',  ( -62.09999999999997300, -2.636465585633694264, 0.1493792525119592707 ) ) ;
#29282=DIRECTION ( 'NONE',  ( 0.000000000000000000, 0.9996898646859343485, 0.02490330187381116153 ) ) ;
#29302=CARTESIAN_POINT ( 'NONE',  ( -73.89999999999997726, -2.435524336289708093E-15, 4.607889071584891164E-15 ) ) ;
#29324=CARTESIAN_POINT ( 'NONE',  ( -62.09999999999997300, -2.663342603746559512, -0.2885805439117342108 ) ) ;
#29344=EDGE_LOOP ( 'NONE', ( #24573, #28984, #22218, #25430 ) ) ;
#29347=CARTESIAN_POINT ( 'NONE',  ( -61.14517784068949879, -2.535105743723619742, -0.9343305864993693977 ) ) ;
#29379=EDGE_CURVE ( 'NONE', #1808, #10647, #18716, .T. ) ;
#29390=AXIS2_PLACEMENT_3D ( 'NONE', #11301, #18456, #4183 ) ;
#29391=DIRECTION ( 'NONE',  ( 3.002035892788117459E-16, -0.9996898646859343485, -0.02490330187381123786 ) ) ;
#29407=EDGE_CURVE ( 'NONE', #30896, #31077, #29136, .T. ) ;
#29424=CARTESIAN_POINT ( 'NONE',  ( -62.06710100716625789, -2.637635658083895329, 0.1963493119579511614 ) ) ;
#29434=DIRECTION ( 'NONE',  ( 1.000000000000000000, 3.053848253006669023E-16, -2.042510438544995415E-16 ) ) ;
#29435=DIRECTION ( 'NONE',  ( 0.000000000000000000, -0.9996898646859343485, -0.02490330187381123786 ) ) ;
#29436=ORIENTED_EDGE ( 'NONE', *, *, #20534, .F. ) ;
#29446=VERTEX_POINT ( 'NONE', #31037 ) ;
#29448=VERTEX_POINT ( 'NONE', #16480 ) ;
#29457=CARTESIAN_POINT ( 'NONE',  ( -61.35212809946285972, -2.542122018907453374, -0.7980057954928057029 ) ) ;
#29459=CARTESIAN_POINT ( 'NONE',  ( -62.09559345744012404, -2.519030794919479010, 0.1735854400584113666 ) ) ;
#29470=CARTESIAN_POINT ( 'NONE',  ( -61.38468220210111070, -2.652782842985662803, 0.4917085785661312047 ) ) ;
#29473=DIRECTION ( 'NONE',  ( -1.000000000000000000, -3.053848253006669023E-16, 2.042510438544995415E-16 ) ) ;
#29486=ORIENTED_EDGE ( 'NONE', *, *, #19545, .T. ) ;
#29507=CARTESIAN_POINT ( 'NONE',  ( -62.09999999999997300, -2.509076856576755166, -0.2831785779091364752 ) ) ;
#29516=DIRECTION ( 'NONE',  ( -1.000000000000000000, -3.053848253006669023E-16, 2.042510438544995415E-16 ) ) ;
#29517=ORIENTED_EDGE ( 'NONE', *, *, #10051, .F. ) ;
#29533=DIRECTION ( 'NONE',  ( -1.000000000000000000, -3.053848253006669023E-16, 2.042510438544995415E-16 ) ) ;
#29551=ADVANCED_FACE ( 'NONE', ( #18675 ), #27715, .T. ) ;
#29552=VERTEX_POINT ( 'NONE', #11065 ) ;
#29561=DIRECTION ( 'NONE',  ( 1.000000000000000000, 3.053848253006669023E-16, -2.042510438544995415E-16 ) ) ;
#29573=CARTESIAN_POINT ( 'NONE',  ( -60.61746561950877066, -2.507927281935157904, 0.9671963751729155678 ) ) ;
#29582=CARTESIAN_POINT ( 'NONE',  ( -73.84999999999996589, -1.301636140808608788, -0.03242509391109853201 ) ) ;
#29620=CARTESIAN_POINT ( 'NONE',  ( -67.34999999999998010, 2.149333209074759221, 0.05354209902869744991 ) ) ;
#29664=CIRCLE ( 'NONE', #9467, 2.750000000000000444 ) ;
#29667=CYLINDRICAL_SURFACE ( 'NONE', #5369, 0.05000000000000002359 ) ;
#29675=ORIENTED_EDGE ( 'NONE', *, *, #12439, .T. ) ;
#29679=CIRCLE ( 'NONE', #30677, 0.04999999999999998890 ) ;
#29683=CARTESIAN_POINT ( 'NONE',  ( -61.35992329370969856, -2.592651747033025700, 0.6797782513837864471 ) ) ;
#29687=ORIENTED_EDGE ( 'NONE', *, *, #1892, .F. ) ;
#29703=LINE ( 'NONE', #3582, #22598 ) ;
#29708=CARTESIAN_POINT ( 'NONE',  ( -61.36283610645477182, -2.650144964772158218, 0.5164607106961540683 ) ) ;
#29712=DIRECTION ( 'NONE',  ( -1.000000000000000000, -3.053848253006669023E-16, 2.042510438544995415E-16 ) ) ;
#29729=CARTESIAN_POINT ( 'NONE',  ( -60.59999999999997300, -2.421197128371385343, -1.061873357074170077 ) ) ;
#29740=ORIENTED_EDGE ( 'NONE', *, *, #6388, .F. ) ;
#29745=( BOUNDED_CURVE ( )  B_SPLINE_CURVE ( 3, ( #27909, #15728, #3680, #13319 ),
 .UNSPECIFIED., .F., .T. ) 
 B_SPLINE_CURVE_WITH_KNOTS ( ( 4, 4 ),
 ( 4.816328208040331127, 4.921019051201621863 ),
 .UNSPECIFIED. ) 
 CURVE ( )  GEOMETRIC_REPRESENTATION_ITEM ( )  RATIONAL_B_SPLINE_CURVE ( ( 1.000000000000000000, 0.9990868608118155247, 0.9990868608118155247, 1.000000000000000000 ) ) 
 REPRESENTATION_ITEM ( '' )  );
#29784=CARTESIAN_POINT ( 'NONE',  ( -62.09962743728070933, -2.519971547655114108, 0.1593117589168163151 ) ) ;
#29785=DIRECTION ( 'NONE',  ( -1.000000000000000000, -3.053848253006669023E-16, 2.042510438544995415E-16 ) ) ;
#29790=DIRECTION ( 'NONE',  ( 1.000000000000000000, 3.053848253006669023E-16, -2.042510438544995415E-16 ) ) ;
#29796=CARTESIAN_POINT ( 'NONE',  ( -61.39046581447303197, -2.653474656127174924, 0.4959525385592167823 ) ) ;
#29798=CIRCLE ( 'NONE', #22747, 2.525000000000001243 ) ;
#29890=CARTESIAN_POINT ( 'NONE',  ( -62.29999999999998295, 1.106939637198029038E-15, 2.238576962872695299E-15 ) ) ;
#29893=CARTESIAN_POINT ( 'NONE',  ( -62.06710100716625789, -2.624587610216423172, -0.3274367013645053115 ) ) ;
#29911=ORIENTED_EDGE ( 'NONE', *, *, #18414, .T. ) ;
#29916=DIRECTION ( 'NONE',  ( 0.000000000000000000, 0.9996898646859344595, 0.02490330187381124133 ) ) ;
#29919=FACE_OUTER_BOUND ( 'NONE', #12384, .T. ) ;
#29923=SHAPE_REPRESENTATION ( 'Twister Head', ( #9018 ), #15625 ) ;
#29952=CARTESIAN_POINT ( 'NONE',  ( -60.61395381780661751, -2.454888324004492972, -1.087441295755433579 ) ) ;
#29956=ORIENTED_EDGE ( 'NONE', *, *, #16946, .T. ) ;
#29961=CARTESIAN_POINT ( 'NONE',  ( -73.90999999999998238, -2.438578184542714499E-15, 4.609931582023435380E-15 ) ) ;
#29998=CARTESIAN_POINT ( 'NONE',  ( -61.34999999999997300, -2.565134197206211386, 0.6652717868084008224 ) ) ;
#30026=VERTEX_POINT ( 'NONE', #25903 ) ;
#30073=AXIS2_PLACEMENT_3D ( 'NONE', #19353, #4757, #30901 ) ;
#30076=CARTESIAN_POINT ( 'NONE',  ( -74.39999999999997726, -2.588216748940040213E-15, 4.710014593512140639E-15 ) ) ;
#30084=CARTESIAN_POINT ( 'NONE',  ( -61.09509470490394278, -2.484918463451591730, -0.8819564647444799732 ) ) ;
#30094=CARTESIAN_POINT ( 'NONE',  ( -60.64959257988790853, -2.458630613964993383, -1.115856434191108359 ) ) ;
#30114=CARTESIAN_POINT ( 'NONE',  ( -61.34999999999997300, -2.528827883897363904, -0.7921676171260561006 ) ) ;
#30118=AXIS2_PLACEMENT_3D ( 'NONE', #25995, #28228, #9068 ) ;
#30127=DIRECTION ( 'NONE',  ( -2.117927888850090838E-16, 0.02490330187381123786, -0.9996898646859343485 ) ) ;
#30131=EDGE_LOOP ( 'NONE', ( #16057, #27613, #2700, #23782, #761 ) ) ;
#30141=CARTESIAN_POINT ( 'NONE',  ( -61.35193852616566090, -2.578113109134980707, 0.6701466704936713814 ) ) ;
#30167=AXIS2_PLACEMENT_3D ( 'NONE', #4270, #30730, #18862 ) ;
#30178=ORIENTED_EDGE ( 'NONE', *, *, #10400, .F. ) ;
#30202=DIRECTION ( 'NONE',  ( 1.000000000000000000, 3.053848253006669023E-16, -2.042510438544995415E-16 ) ) ;
#30204=VECTOR ( 'NONE', #28020, 999.9999999999998863 ) ;
#30213=ADVANCED_FACE ( 'NONE', ( #15274, #7823 ), #7539, .T. ) ;
#30216=LINE ( 'NONE', #8360, #26078 ) ;
#30264=CARTESIAN_POINT ( 'NONE',  ( -60.62155403265821718, -2.458719867916568269, -1.094860189600118439 ) ) ;
#30265=ORIENTED_EDGE ( 'NONE', *, *, #22364, .F. ) ;
#30292=DIRECTION ( 'NONE',  ( -3.002035892788117952E-16, 0.9996898646859344595, 0.02490330187381124133 ) ) ;
#30300=DIRECTION ( 'NONE',  ( -1.000000000000000000, -3.053848253006669023E-16, 2.042510438544995415E-16 ) ) ;
#30317=CARTESIAN_POINT ( 'NONE',  ( -62.09999999999997300, -2.737615117699082834, 0.2585595776647297561 ) ) ;
#30371=VERTEX_POINT ( 'NONE', #9179 ) ;
#30376=ORIENTED_EDGE ( 'NONE', *, *, #16787, .T. ) ;
#30382=( BOUNDED_SURFACE ( )  B_SPLINE_SURFACE ( 3, 2, ( 
 ( #10102, #29263, #10248 ),
 ( #14834, #17543, #5504 ),
 ( #21697, #26563, #17233 ),
 ( #26741, #5330, #9654 ) ),
 .UNSPECIFIED., .F., .F., .F. ) 
 B_SPLINE_SURFACE_WITH_KNOTS ( ( 4, 4 ),
 ( 3, 3 ),
 ( 4.828596150434655954, 4.929762646526004488 ),
 ( 0.000000000000000000, 1.000000000000000000 ),
 .UNSPECIFIED. ) 
 GEOMETRIC_REPRESENTATION_ITEM ( )  RATIONAL_B_SPLINE_SURFACE ( (
 ( 1.000000000000000000, 0.6674753128239091504, 1.000000000000000000),
 ( 1.000000000000000000, 0.6556866267091900902, 1.000000000000000000),
 ( 1.000000000000000000, 0.6436549836476661568, 1.000000000000000000),
 ( 1.000000000000000000, 0.6314033579135635010, 1.000000000000000000) ) ) 
 REPRESENTATION_ITEM ( '' )  SURFACE ( )  );
#30402=CARTESIAN_POINT ( 'NONE',  ( -62.06598287454225726, -2.648582569373490347, -0.3347775276703480740 ) ) ;
#30418=ADVANCED_FACE ( 'NONE', ( #2670 ), #26686, .T. ) ;
#30421=ORIENTED_EDGE ( 'NONE', *, *, #20266, .F. ) ;
#30423=ORIENTED_EDGE ( 'NONE', *, *, #5441, .T. ) ;
#30432=SURFACE_STYLE_FILL_AREA ( #18745 ) ;
#30449=EDGE_LOOP ( 'NONE', ( #31295, #14861, #10530, #8071 ) ) ;
#30459=CARTESIAN_POINT ( 'NONE',  ( -61.34999999999997300, -2.600201727571727517, 0.4583662226975599441 ) ) ;
#30465=EDGE_CURVE ( 'NONE', #14068, #30753, #26569, .T. ) ;
#30470=CARTESIAN_POINT ( 'NONE',  ( -60.83824777938932726, -2.565600044710441008, 0.8496564960046820714 ) ) ;
#30493=CYLINDRICAL_SURFACE ( 'NONE', #31266, 1.250000000000000222 ) ;
#30509=B_SPLINE_CURVE_WITH_KNOTS ( 'NONE', 3,
 ( #29424, #7137, #7733, #28969, #12638, #4733, #24065, #2378, #21717, #8, #19333, #7277, #16947, #26591, #4901, #14566, #24230, #2540, #12191 ),
 .UNSPECIFIED., .F., .F.,
 ( 4, 3, 3, 3, 3, 3, 4 ),
 ( 0.000000000000000000, 1.590918590077522167E-05, 3.217562587127302352E-05, 4.946895718673912572E-05, 6.849224166005159653E-05, 8.924830576836555271E-05, 9.321254545577940852E-05 ),
 .UNSPECIFIED. ) ;
#30514=ORIENTED_EDGE ( 'NONE', *, *, #17955, .F. ) ;
#30544=DIRECTION ( 'NONE',  ( 0.000000000000000000, -0.9996898646859344595, -0.02490330187381124480 ) ) ;
#30553=CARTESIAN_POINT ( 'NONE',  ( -62.06710100716625789, -2.624587610216423172, -0.3274367013645053115 ) ) ;
#30559=CONICAL_SURFACE ( 'NONE', #24509, 1.600000000000000533, 0.7853981633974497223 ) ;
#30585=FILL_AREA_STYLE_COLOUR ( '', #23124 ) ;
#30612=ORIENTED_EDGE ( 'NONE', *, *, #17955, .T. ) ;
#30617=ORIENTED_EDGE ( 'NONE', *, *, #19294, .T. ) ;
#30623=CARTESIAN_POINT ( 'NONE',  ( -62.09999999999997300, -2.636465585633694264, 0.1493792525119592707 ) ) ;
#30641=CIRCLE ( 'NONE', #21068, 2.700000000000000178 ) ;
#30655=FACE_OUTER_BOUND ( 'NONE', #2443, .T. ) ;
#30658=CARTESIAN_POINT ( 'NONE',  ( -60.49999999999997868, 1.656632322739229403E-15, 1.870925083934595927E-15 ) ) ;
#30673=CARTESIAN_POINT ( 'NONE',  ( -62.29999999999998295, 2.799131621120617641, 0.06972924524667370449 ) ) ;
#30677=AXIS2_PLACEMENT_3D ( 'NONE', #28897, #23842, #2459 ) ;
#30681=CARTESIAN_POINT ( 'NONE',  ( -64.31974649313019654, -2.248654970328749947, -0.05601630617084708830 ) ) ;
#30682=EDGE_LOOP ( 'NONE', ( #25596, #28438, #15883, #6798 ) ) ;
#30696=ADVANCED_FACE ( 'NONE', ( #11191 ), #30493, .T. ) ;
#30700=CLOSED_SHELL ( 'NONE', ( #31104, #9962, #15328, #17524, #8467, #6327, #9305, #10362, #26400, #18998, #866, #10053, #30696, #13331, #8969, #22611, #9463, #27180, #14786, #7281, #15402, #20357, #30213, #21839, #1217, #15640, #13212, #8701, #5387, #4220, #7739, #4783, #5454, #13136, #5114, #3783, #27666, #20108, #15662, #3979, #12720, #21834, #8282, #17269, #9640, #21643, #29551, #27167, #11902, #25734, #24059, #10556, #30418, #6883, #26691, #1473, #1702, #15053, #6008, #5151, #7554, #3775, #23815, #20060, #20677, #6185, #16817, #1234, #18620 ) ) ;
#30714=CARTESIAN_POINT ( 'NONE',  ( -62.09999999999998010, -2.742892450101797053, 0.2063307189744075232 ) ) ;
#30730=DIRECTION ( 'NONE',  ( 3.002035892788116966E-16, -0.9996898646859343485, -0.02490330187381123786 ) ) ;
#30743=AXIS2_PLACEMENT_3D ( 'NONE', #9461, #9145, #24013 ) ;
#30753=VERTEX_POINT ( 'NONE', #1676 ) ;
#30757=CARTESIAN_POINT ( 'NONE',  ( -62.09999999999997300, -2.520404473256288469, 0.1522704540930145123 ) ) ;
#30760=CARTESIAN_POINT ( 'NONE',  ( -61.10430241999912937, -2.555382569520581626, -0.8803594241308302371 ) ) ;
#30762=( BOUNDED_CURVE ( )  B_SPLINE_CURVE ( 3, ( #3954, #23286, #29347, #7658 ),
 .UNSPECIFIED., .F., .T. ) 
 B_SPLINE_CURVE_WITH_KNOTS ( ( 4, 4 ),
 ( 1.169545686397452711, 1.279118582711132435 ),
 .UNSPECIFIED. ) 
 CURVE ( )  GEOMETRIC_REPRESENTATION_ITEM ( )  RATIONAL_B_SPLINE_CURVE ( ( 1.000000000000000000, 0.9989997319336324511, 0.9989997319336324511, 1.000000000000000000 ) ) 
 REPRESENTATION_ITEM ( '' )  );
#30767=FACE_OUTER_BOUND ( 'NONE', #13937, .T. ) ;
#30780=ORIENTED_EDGE ( 'NONE', *, *, #15008, .T. ) ;
#30790=DIRECTION ( 'NONE',  ( -1.000000000000000000, -3.053848253006669023E-16, 2.042510438544995415E-16 ) ) ;
#30793=EDGE_CURVE ( 'NONE', #10647, #30371, #13036, .T. ) ;
#30794=DIRECTION ( 'NONE',  ( 0.000000000000000000, 0.9996898646859344595, 0.02490330187381124480 ) ) ;
#30814=ORIENTED_EDGE ( 'NONE', *, *, #12781, .T. ) ;
#30819=DIRECTION ( 'NONE',  ( 2.117927888850091331E-16, -0.02490330187381135929, 0.9996898646859343485 ) ) ;
#30821=DIRECTION ( 'NONE',  ( -1.000000000000000000, -3.053848253006669023E-16, 2.042510438544995415E-16 ) ) ;
#30824=VECTOR ( 'NONE', #2039, 1000.000000000000000 ) ;
#30841=CARTESIAN_POINT ( 'NONE',  ( -62.14999999999998437, -2.799131621120614977, -0.06972924524666890278 ) ) ;
#30864=ORIENTED_EDGE ( 'NONE', *, *, #8115, .F. ) ;
#30870=CARTESIAN_POINT ( 'NONE',  ( -62.09999999999998010, -2.636465585633694264, 0.1493792525119599646 ) ) ;
#30880=DIRECTION ( 'NONE',  ( 0.000000000000000000, 0.9996898646859344595, 0.02490330187381124827 ) ) ;
#30889=CARTESIAN_POINT ( 'NONE',  ( -62.05200726403181477, -2.672099260701759516, -0.3872133491583026887 ) ) ;
#30896=VERTEX_POINT ( 'NONE', #13209 ) ;
#30897=ORIENTED_EDGE ( 'NONE', *, *, #21399, .T. ) ;
#30901=DIRECTION ( 'NONE',  ( 0.000000000000000000, 0.9996898646859343485, 0.02490330187381123786 ) ) ;
#30919=EDGE_CURVE ( 'NONE', #2594, #21812, #11029, .T. ) ;
#30925=EDGE_CURVE ( 'NONE', #12162, #7685, #23182, .T. ) ;
#30944=VERTEX_POINT ( 'NONE', #6715 ) ;
#30947=CARTESIAN_POINT ( 'NONE',  ( -73.89999999999997726, -2.435524336289708093E-15, 4.607889071584891164E-15 ) ) ;
#30967=EDGE_LOOP ( 'NONE', ( #25506, #26319 ) ) ;
#31016=CARTESIAN_POINT ( 'NONE',  ( -61.36062461429197157, -2.612524402084908548, -0.6029330766772686978 ) ) ;
#31019=ORIENTED_EDGE ( 'NONE', *, *, #13839, .F. ) ;
#31029=AXIS2_PLACEMENT_3D ( 'NONE', #22260, #12410, #17331 ) ;
#31037=CARTESIAN_POINT ( 'NONE',  ( -73.90999999999998238, -1.249612330857420517, -0.03112912734225924127 ) ) ;
#31047=B_SPLINE_CURVE_WITH_KNOTS ( 'NONE', 3,
 ( #15439, #27468, #8163, #29998 ),
 .UNSPECIFIED., .F., .F.,
 ( 4, 4 ),
 ( 0.000000000000000000, 1.346394374510334621E-05 ),
 .UNSPECIFIED. ) ;
#31065=CARTESIAN_POINT ( 'NONE',  ( -60.59999999999998010, -2.292917048100124866, -1.057429151542457868 ) ) ;
#31068=EDGE_CURVE ( 'NONE', #19690, #28771, #27713, .T. ) ;
#31077=VERTEX_POINT ( 'NONE', #23831 ) ;
#31090=DIRECTION ( 'NONE',  ( 0.000000000000000000, -0.9892893632948467353, -0.1459676528264966522 ) ) ;
#31104=ADVANCED_FACE ( 'NONE', ( #17020 ), #7655, .F. ) ;
#31124=AXIS2_PLACEMENT_3D ( 'NONE', #17606, #17436, #27251 ) ;
#31129=AXIS2_PLACEMENT_3D ( 'NONE', #4184, #13822, #14164 ) ;
#31137=FACE_OUTER_BOUND ( 'NONE', #26660, .T. ) ;
#31167=CARTESIAN_POINT ( 'NONE',  ( -62.39999999999998437, -2.699162634652021886, -0.06723891505928761281 ) ) ;
#31196=CARTESIAN_POINT ( 'NONE',  ( -61.82794808878163906, -2.629646814551887424, 0.2836198699518600597 ) ) ;
#31213=CARTESIAN_POINT ( 'NONE',  ( -61.39999999999998437, 1.381785979968628826E-15, 2.054751023403646402E-15 ) ) ;
#31220=ORIENTED_EDGE ( 'NONE', *, *, #16984, .T. ) ;
#31247=DIRECTION ( 'NONE',  ( 1.000000000000000000, 3.053848253006669023E-16, -2.042510438544995415E-16 ) ) ;
#31266=AXIS2_PLACEMENT_3D ( 'NONE', #25439, #8797, #4215 ) ;
#31272=ORIENTED_EDGE ( 'NONE', *, *, #22424, .T. ) ;
#31295=ORIENTED_EDGE ( 'NONE', *, *, #9177, .T. ) ;
#31300=FACE_OUTER_BOUND ( 'NONE', #26774, .T. ) ;
ENDSEC;
END-ISO-10303-21;
